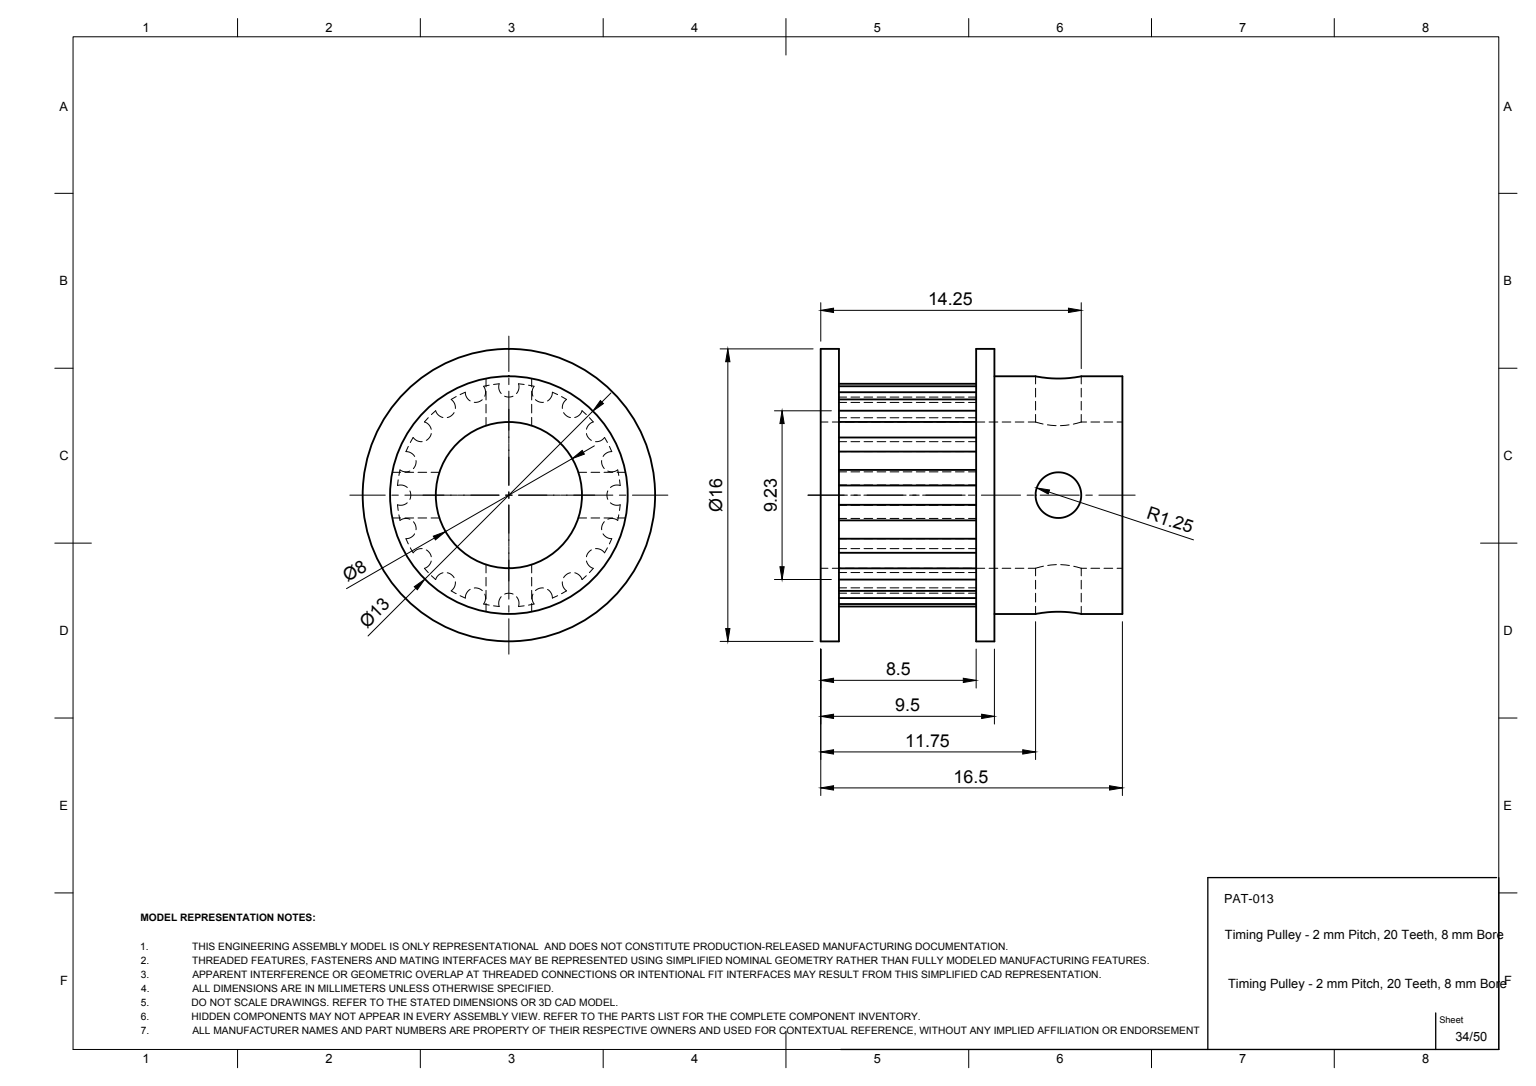
ISO-10303-21;
HEADER;
/* Generated by software containing ST-Developer
 * from STEP Tools, Inc. (www.steptools.com) 
 */

FILE_DESCRIPTION(
/* description */ ('Belt-driven linear axis on 2020 extrusion'),
/* implementation_level */ '2;1');

FILE_NAME(
/* name */ 'Timing Pulley - 2 mm Pitch, 20 Teeth, 8 mm Bore.step',
/* time_stamp */ '2026-10-28T03:26:09-07:00',
/* author */ (''),
/* organization */ (''),
/* preprocessor_version */ 'ST-DEVELOPER v20.2',
/* originating_system */ 'Autodesk Translation Framework v15.17.0.0',
/* authorisation */ '');

FILE_SCHEMA (('AUTOMOTIVE_DESIGN { 1 0 10303 214 3 1 1 }'));
ENDSEC;

DATA;
#10=MECHANICAL_DESIGN_GEOMETRIC_PRESENTATION_REPRESENTATION('',(#655),#20096);
#459=B_SPLINE_CURVE_WITH_KNOTS('',3,(#18624,#18625,#18626,#18627,#18628,
#18629,#18630,#18631,#18632,#18633),.UNSPECIFIED.,.F.,.F.,(4,2,2,2,4),(0.566550474129931,
0.613761886174531,0.66097329821913,0.708186965196186,0.755400632173242),
 .UNSPECIFIED.);
#460=B_SPLINE_CURVE_WITH_KNOTS('',3,(#18635,#18636,#18637,#18638,#18639,
#18640,#18641,#18642,#18643,#18644,#18645,#18646,#18647,#18648,#18649,#18650,
#18651,#18652),.UNSPECIFIED.,.F.,.F.,(4,2,2,2,2,2,2,2,4),(0.18885015804331,
0.23606157008791,0.283272982132509,0.330486649109565,0.377700316086621,
0.424913983063677,0.472127650040732,0.519339062085332,0.566550474129931),
 .UNSPECIFIED.);
#461=B_SPLINE_CURVE_WITH_KNOTS('',3,(#18653,#18654,#18655,#18656,#18657,
#18658,#18659,#18660,#18661,#18662),.UNSPECIFIED.,.F.,.F.,(4,2,2,2,4),(0.755400632173242,
0.802614299150298,0.849827966127353,0.897039378171953,0.944250790216552),
 .UNSPECIFIED.);
#462=B_SPLINE_CURVE_WITH_KNOTS('',3,(#18666,#18667,#18668,#18669,#18670,
#18671,#18672,#18673,#18674,#18675),.UNSPECIFIED.,.F.,.F.,(4,2,2,2,4),(0.189723673274825,
0.237146208024627,0.28456874277443,0.33200804466204,0.37944734654965),
 .UNSPECIFIED.);
#463=B_SPLINE_CURVE_WITH_KNOTS('',3,(#18677,#18678,#18679,#18680,#18681,
#18682,#18683,#18684,#18685,#18686),.UNSPECIFIED.,.F.,.F.,(4,2,2,2,4),(0.,
0.0474393018876097,0.0948786037752193,0.142301138525022,0.189723673274825),
 .UNSPECIFIED.);
#464=B_SPLINE_CURVE_WITH_KNOTS('',3,(#18688,#18689,#18690,#18691,#18692,
#18693,#18694,#18695,#18696,#18697),.UNSPECIFIED.,.F.,.F.,(4,2,2,2,4),(0.569171019824474,
0.616593554574277,0.66401608932408,0.711455391211689,0.758894693099299),
 .UNSPECIFIED.);
#465=B_SPLINE_CURVE_WITH_KNOTS('',3,(#18698,#18699,#18700,#18701,#18702,
#18703,#18704,#18705,#18706,#18707),.UNSPECIFIED.,.F.,.F.,(4,2,2,2,4),(0.37944734654965,
0.426886648437259,0.474325950324869,0.521748485074671,0.569171019824474),
 .UNSPECIFIED.);
#466=B_SPLINE_CURVE_WITH_KNOTS('',3,(#18711,#18712,#18713,#18714,#18715,
#18716,#18717,#18718,#18719,#18720,#18721,#18722,#18723,#18724,#18725,#18726,
#18727,#18728),.UNSPECIFIED.,.F.,.F.,(4,2,2,2,2,2,2,2,4),(0.,0.0474393018876097,
0.0948786037752194,0.142301138525022,0.189723673274825,0.237146208024628,
0.28456874277443,0.33200804466204,0.37944734654965),.UNSPECIFIED.);
#467=B_SPLINE_CURVE_WITH_KNOTS('',3,(#18729,#18730,#18731,#18732,#18733,
#18734,#18735,#18736,#18737,#18738,#18739,#18740,#18741,#18742,#18743,#18744,
#18745,#18746),.UNSPECIFIED.,.F.,.F.,(4,2,2,2,2,2,2,2,4),(0.37944734654965,
0.426886648437259,0.474325950324869,0.521748485074672,0.569171019824474,
0.616593554574277,0.66401608932408,0.711455391211689,0.758894693099299),
 .UNSPECIFIED.);
#468=B_SPLINE_CURVE_WITH_KNOTS('',3,(#18750,#18751,#18752,#18753,#18754,
#18755,#18756,#18757,#18758,#18759),.UNSPECIFIED.,.F.,.F.,(4,2,2,2,4),(0.566550474129931,
0.613761886174531,0.66097329821913,0.708186965196186,0.755400632173242),
 .UNSPECIFIED.);
#469=B_SPLINE_CURVE_WITH_KNOTS('',3,(#18761,#18762,#18763,#18764,#18765,
#18766,#18767,#18768,#18769,#18770,#18771,#18772,#18773,#18774,#18775,#18776,
#18777,#18778),.UNSPECIFIED.,.F.,.F.,(4,2,2,2,2,2,2,2,4),(0.188850158043311,
0.23606157008791,0.283272982132509,0.330486649109565,0.377700316086621,
0.424913983063677,0.472127650040733,0.519339062085332,0.566550474129931),
 .UNSPECIFIED.);
#470=B_SPLINE_CURVE_WITH_KNOTS('',3,(#18779,#18780,#18781,#18782,#18783,
#18784,#18785,#18786,#18787,#18788),.UNSPECIFIED.,.F.,.F.,(4,2,2,2,4),(0.755400632173242,
0.802614299150298,0.849827966127354,0.897039378171953,0.944250790216552),
 .UNSPECIFIED.);
#471=B_SPLINE_CURVE_WITH_KNOTS('',3,(#18798,#18799,#18800,#18801,#18802,
#18803,#18804,#18805,#18806,#18807,#18808,#18809,#18810,#18811,#18812,#18813,
#18814,#18815),.UNSPECIFIED.,.F.,.F.,(4,2,2,2,2,2,2,2,4),(0.18885015804331,
0.23606157008791,0.283272982132509,0.330486649109565,0.377700316086621,
0.424913983063677,0.472127650040732,0.519339062085332,0.566550474129931),
 .UNSPECIFIED.);
#472=B_SPLINE_CURVE_WITH_KNOTS('',3,(#18817,#18818,#18819,#18820,#18821,
#18822,#18823,#18824,#18825,#18826),.UNSPECIFIED.,.F.,.F.,(4,2,2,2,4),(0.566550474129931,
0.613761886174531,0.66097329821913,0.708186965196186,0.755400632173242),
 .UNSPECIFIED.);
#473=B_SPLINE_CURVE_WITH_KNOTS('',3,(#18827,#18828,#18829,#18830,#18831,
#18832,#18833,#18834,#18835,#18836),.UNSPECIFIED.,.F.,.F.,(4,2,2,2,4),(0.755400632173242,
0.802614299150298,0.849827966127353,0.897039378171953,0.944250790216552),
 .UNSPECIFIED.);
#474=B_SPLINE_CURVE_WITH_KNOTS('',3,(#18839,#18840,#18841,#18842,#18843,
#18844,#18845,#18846,#18847,#18848,#18849,#18850,#18851,#18852,#18853,#18854,
#18855,#18856),.UNSPECIFIED.,.F.,.F.,(4,2,2,2,2,2,2,2,4),(0.188850158043311,
0.23606157008791,0.283272982132509,0.330486649109565,0.377700316086621,
0.424913983063677,0.472127650040733,0.519339062085332,0.566550474129932),
 .UNSPECIFIED.);
#475=B_SPLINE_CURVE_WITH_KNOTS('',3,(#18858,#18859,#18860,#18861,#18862,
#18863,#18864,#18865,#18866,#18867),.UNSPECIFIED.,.F.,.F.,(4,2,2,2,4),(0.566550474129932,
0.613761886174531,0.66097329821913,0.708186965196186,0.755400632173242),
 .UNSPECIFIED.);
#476=B_SPLINE_CURVE_WITH_KNOTS('',3,(#18868,#18869,#18870,#18871,#18872,
#18873,#18874,#18875,#18876,#18877),.UNSPECIFIED.,.F.,.F.,(4,2,2,2,4),(0.755400632173242,
0.802614299150298,0.849827966127354,0.897039378171953,0.944250790216552),
 .UNSPECIFIED.);
#477=B_SPLINE_CURVE_WITH_KNOTS('',3,(#18882,#18883,#18884,#18885,#18886,
#18887,#18888,#18889,#18890,#18891,#18892,#18893,#18894,#18895,#18896,#18897,
#18898,#18899),.UNSPECIFIED.,.F.,.F.,(4,2,2,2,2,2,2,2,4),(0.,0.0474393018876097,
0.0948786037752193,0.142301138525022,0.189723673274825,0.237146208024627,
0.28456874277443,0.33200804466204,0.37944734654965),.UNSPECIFIED.);
#478=B_SPLINE_CURVE_WITH_KNOTS('',3,(#18900,#18901,#18902,#18903,#18904,
#18905,#18906,#18907,#18908,#18909,#18910,#18911,#18912,#18913,#18914,#18915,
#18916,#18917),.UNSPECIFIED.,.F.,.F.,(4,2,2,2,2,2,2,2,4),(0.37944734654965,
0.426886648437259,0.474325950324869,0.521748485074672,0.569171019824474,
0.616593554574277,0.66401608932408,0.711455391211689,0.758894693099299),
 .UNSPECIFIED.);
#479=B_SPLINE_CURVE_WITH_KNOTS('',3,(#18921,#18922,#18923,#18924,#18925,
#18926,#18927,#18928,#18929,#18930,#18931,#18932,#18933,#18934,#18935,#18936,
#18937,#18938),.UNSPECIFIED.,.F.,.F.,(4,2,2,2,2,2,2,2,4),(0.,0.0474393018876097,
0.0948786037752194,0.142301138525022,0.189723673274825,0.237146208024627,
0.28456874277443,0.33200804466204,0.37944734654965),.UNSPECIFIED.);
#480=B_SPLINE_CURVE_WITH_KNOTS('',3,(#18939,#18940,#18941,#18942,#18943,
#18944,#18945,#18946,#18947,#18948,#18949,#18950,#18951,#18952,#18953,#18954,
#18955,#18956),.UNSPECIFIED.,.F.,.F.,(4,2,2,2,2,2,2,2,4),(0.37944734654965,
0.426886648437259,0.474325950324869,0.521748485074672,0.569171019824474,
0.616593554574277,0.66401608932408,0.711455391211689,0.758894693099299),
 .UNSPECIFIED.);
#553=SHAPE_REPRESENTATION_RELATIONSHIP('SRR','None',#20352,#599);
#599=ADVANCED_BREP_SHAPE_REPRESENTATION('',(#710),#20083);
#655=STYLED_ITEM('',(#20664),#710);
#710=MANIFOLD_SOLID_BREP('Body1',#10969);
#851=FACE_BOUND('',#2438,.T.);
#852=FACE_BOUND('',#2439,.T.);
#853=FACE_BOUND('',#2440,.T.);
#854=FACE_BOUND('',#2444,.T.);
#855=FACE_BOUND('',#2445,.T.);
#856=FACE_BOUND('',#2446,.T.);
#857=FACE_BOUND('',#2448,.T.);
#858=FACE_BOUND('',#2450,.T.);
#859=FACE_BOUND('',#2453,.T.);
#860=FACE_BOUND('',#2455,.T.);
#861=FACE_BOUND('',#2458,.T.);
#1144=PLANE('',#12331);
#1145=PLANE('',#12332);
#1146=PLANE('',#12376);
#1147=PLANE('',#12377);
#1148=PLANE('',#12421);
#1680=FACE_OUTER_BOUND('',#2435,.T.);
#1681=FACE_OUTER_BOUND('',#2436,.T.);
#1682=FACE_OUTER_BOUND('',#2437,.T.);
#1683=FACE_OUTER_BOUND('',#2441,.T.);
#1684=FACE_OUTER_BOUND('',#2442,.T.);
#1685=FACE_OUTER_BOUND('',#2443,.T.);
#1686=FACE_OUTER_BOUND('',#2447,.T.);
#1687=FACE_OUTER_BOUND('',#2449,.T.);
#1688=FACE_OUTER_BOUND('',#2451,.T.);
#1689=FACE_OUTER_BOUND('',#2452,.T.);
#1690=FACE_OUTER_BOUND('',#2454,.T.);
#1691=FACE_OUTER_BOUND('',#2456,.T.);
#1692=FACE_OUTER_BOUND('',#2457,.T.);
#1693=FACE_OUTER_BOUND('',#2459,.T.);
#1694=FACE_OUTER_BOUND('',#2460,.T.);
#1695=FACE_OUTER_BOUND('',#2461,.T.);
#1696=FACE_OUTER_BOUND('',#2462,.T.);
#1697=FACE_OUTER_BOUND('',#2463,.T.);
#1698=FACE_OUTER_BOUND('',#2464,.T.);
#1699=FACE_OUTER_BOUND('',#2465,.T.);
#1700=FACE_OUTER_BOUND('',#2466,.T.);
#1701=FACE_OUTER_BOUND('',#2467,.T.);
#1702=FACE_OUTER_BOUND('',#2468,.T.);
#1703=FACE_OUTER_BOUND('',#2469,.T.);
#1704=FACE_OUTER_BOUND('',#2470,.T.);
#1705=FACE_OUTER_BOUND('',#2471,.T.);
#1706=FACE_OUTER_BOUND('',#2472,.T.);
#1707=FACE_OUTER_BOUND('',#2473,.T.);
#1708=FACE_OUTER_BOUND('',#2474,.T.);
#1709=FACE_OUTER_BOUND('',#2475,.T.);
#1710=FACE_OUTER_BOUND('',#2476,.T.);
#1711=FACE_OUTER_BOUND('',#2477,.T.);
#1712=FACE_OUTER_BOUND('',#2478,.T.);
#1713=FACE_OUTER_BOUND('',#2479,.T.);
#1714=FACE_OUTER_BOUND('',#2480,.T.);
#1715=FACE_OUTER_BOUND('',#2481,.T.);
#1716=FACE_OUTER_BOUND('',#2482,.T.);
#1717=FACE_OUTER_BOUND('',#2483,.T.);
#1718=FACE_OUTER_BOUND('',#2484,.T.);
#1719=FACE_OUTER_BOUND('',#2485,.T.);
#1720=FACE_OUTER_BOUND('',#2486,.T.);
#1721=FACE_OUTER_BOUND('',#2487,.T.);
#1722=FACE_OUTER_BOUND('',#2488,.T.);
#1723=FACE_OUTER_BOUND('',#2489,.T.);
#1724=FACE_OUTER_BOUND('',#2490,.T.);
#1725=FACE_OUTER_BOUND('',#2491,.T.);
#1726=FACE_OUTER_BOUND('',#2492,.T.);
#1727=FACE_OUTER_BOUND('',#2493,.T.);
#1728=FACE_OUTER_BOUND('',#2494,.T.);
#1729=FACE_OUTER_BOUND('',#2495,.T.);
#1730=FACE_OUTER_BOUND('',#2496,.T.);
#1731=FACE_OUTER_BOUND('',#2497,.T.);
#1732=FACE_OUTER_BOUND('',#2498,.T.);
#2435=EDGE_LOOP('',(#9133,#9134,#9135,#9136,#9137,#9138,#9139,#9140,#9141));
#2436=EDGE_LOOP('',(#9142,#9143,#9144,#9145,#9146,#9147,#9148));
#2437=EDGE_LOOP('',(#9149,#9150,#9151,#9152,#9153,#9154,#9155,#9156,#9157));
#2438=EDGE_LOOP('',(#9158,#9159,#9160));
#2439=EDGE_LOOP('',(#9161,#9162,#9163));
#2440=EDGE_LOOP('',(#9164,#9165,#9166));
#2441=EDGE_LOOP('',(#9167,#9168,#9169,#9170,#9171,#9172,#9173));
#2442=EDGE_LOOP('',(#9174,#9175,#9176,#9177,#9178,#9179,#9180));
#2443=EDGE_LOOP('',(#9181,#9182,#9183,#9184,#9185,#9186,#9187,#9188,#9189,
#9190));
#2444=EDGE_LOOP('',(#9191,#9192));
#2445=EDGE_LOOP('',(#9193,#9194));
#2446=EDGE_LOOP('',(#9195,#9196));
#2447=EDGE_LOOP('',(#9197));
#2448=EDGE_LOOP('',(#9198));
#2449=EDGE_LOOP('',(#9199));
#2450=EDGE_LOOP('',(#9200,#9201,#9202,#9203,#9204,#9205,#9206,#9207,#9208,
#9209,#9210,#9211,#9212,#9213,#9214,#9215,#9216,#9217,#9218,#9219,#9220,
#9221,#9222,#9223,#9224,#9225,#9226,#9227,#9228,#9229,#9230,#9231,#9232,
#9233,#9234,#9235,#9236,#9237,#9238,#9239));
#2451=EDGE_LOOP('',(#9240,#9241,#9242,#9243));
#2452=EDGE_LOOP('',(#9244));
#2453=EDGE_LOOP('',(#9245));
#2454=EDGE_LOOP('',(#9246));
#2455=EDGE_LOOP('',(#9247,#9248,#9249,#9250,#9251,#9252,#9253,#9254,#9255,
#9256,#9257,#9258,#9259,#9260,#9261,#9262,#9263,#9264,#9265,#9266,#9267,
#9268,#9269,#9270,#9271,#9272,#9273,#9274,#9275,#9276,#9277,#9278,#9279,
#9280,#9281,#9282,#9283,#9284,#9285,#9286));
#2456=EDGE_LOOP('',(#9287,#9288,#9289,#9290));
#2457=EDGE_LOOP('',(#9291));
#2458=EDGE_LOOP('',(#9292));
#2459=EDGE_LOOP('',(#9293,#9294,#9295,#9296));
#2460=EDGE_LOOP('',(#9297,#9298,#9299,#9300));
#2461=EDGE_LOOP('',(#9301,#9302,#9303,#9304));
#2462=EDGE_LOOP('',(#9305,#9306,#9307,#9308));
#2463=EDGE_LOOP('',(#9309,#9310,#9311,#9312));
#2464=EDGE_LOOP('',(#9313,#9314,#9315,#9316));
#2465=EDGE_LOOP('',(#9317,#9318,#9319,#9320));
#2466=EDGE_LOOP('',(#9321,#9322,#9323,#9324));
#2467=EDGE_LOOP('',(#9325,#9326,#9327,#9328));
#2468=EDGE_LOOP('',(#9329,#9330,#9331,#9332));
#2469=EDGE_LOOP('',(#9333,#9334,#9335,#9336));
#2470=EDGE_LOOP('',(#9337,#9338,#9339,#9340));
#2471=EDGE_LOOP('',(#9341,#9342,#9343,#9344));
#2472=EDGE_LOOP('',(#9345,#9346,#9347,#9348));
#2473=EDGE_LOOP('',(#9349,#9350,#9351,#9352));
#2474=EDGE_LOOP('',(#9353,#9354,#9355,#9356));
#2475=EDGE_LOOP('',(#9357,#9358,#9359,#9360));
#2476=EDGE_LOOP('',(#9361,#9362,#9363,#9364));
#2477=EDGE_LOOP('',(#9365,#9366,#9367,#9368));
#2478=EDGE_LOOP('',(#9369,#9370,#9371,#9372));
#2479=EDGE_LOOP('',(#9373,#9374,#9375,#9376));
#2480=EDGE_LOOP('',(#9377,#9378,#9379,#9380));
#2481=EDGE_LOOP('',(#9381,#9382,#9383,#9384));
#2482=EDGE_LOOP('',(#9385,#9386,#9387,#9388));
#2483=EDGE_LOOP('',(#9389,#9390,#9391,#9392));
#2484=EDGE_LOOP('',(#9393,#9394,#9395,#9396));
#2485=EDGE_LOOP('',(#9397,#9398,#9399,#9400));
#2486=EDGE_LOOP('',(#9401,#9402,#9403,#9404));
#2487=EDGE_LOOP('',(#9405,#9406,#9407,#9408));
#2488=EDGE_LOOP('',(#9409,#9410,#9411,#9412));
#2489=EDGE_LOOP('',(#9413,#9414,#9415,#9416));
#2490=EDGE_LOOP('',(#9417,#9418,#9419,#9420));
#2491=EDGE_LOOP('',(#9421,#9422,#9423,#9424));
#2492=EDGE_LOOP('',(#9425,#9426,#9427,#9428));
#2493=EDGE_LOOP('',(#9429,#9430,#9431,#9432));
#2494=EDGE_LOOP('',(#9433,#9434,#9435,#9436));
#2495=EDGE_LOOP('',(#9437,#9438,#9439,#9440));
#2496=EDGE_LOOP('',(#9441,#9442,#9443,#9444));
#2497=EDGE_LOOP('',(#9445,#9446,#9447,#9448));
#2498=EDGE_LOOP('',(#9449,#9450,#9451,#9452));
#3232=LINE('',#18664,#4089);
#3233=LINE('',#18748,#4090);
#3234=LINE('',#18792,#4091);
#3235=LINE('',#18794,#4092);
#3236=LINE('',#18880,#4093);
#3237=LINE('',#18957,#4094);
#3238=LINE('',#18961,#4095);
#3239=LINE('',#18963,#4096);
#3240=LINE('',#19052,#4097);
#3241=LINE('',#19140,#4098);
#3242=LINE('',#19143,#4099);
#3243=LINE('',#19144,#4100);
#3244=LINE('',#19146,#4101);
#3245=LINE('',#19148,#4102);
#3246=LINE('',#19150,#4103);
#3247=LINE('',#19152,#4104);
#3248=LINE('',#19154,#4105);
#3249=LINE('',#19156,#4106);
#3250=LINE('',#19158,#4107);
#3251=LINE('',#19160,#4108);
#3252=LINE('',#19162,#4109);
#3253=LINE('',#19164,#4110);
#3254=LINE('',#19166,#4111);
#3255=LINE('',#19168,#4112);
#3256=LINE('',#19170,#4113);
#3257=LINE('',#19172,#4114);
#3258=LINE('',#19174,#4115);
#3259=LINE('',#19176,#4116);
#3260=LINE('',#19178,#4117);
#3261=LINE('',#19180,#4118);
#3262=LINE('',#19182,#4119);
#3263=LINE('',#19184,#4120);
#3264=LINE('',#19186,#4121);
#3265=LINE('',#19188,#4122);
#3266=LINE('',#19190,#4123);
#3267=LINE('',#19192,#4124);
#3268=LINE('',#19194,#4125);
#3269=LINE('',#19196,#4126);
#3270=LINE('',#19198,#4127);
#3271=LINE('',#19200,#4128);
#3272=LINE('',#19202,#4129);
#3273=LINE('',#19204,#4130);
#3274=LINE('',#19206,#4131);
#3275=LINE('',#19208,#4132);
#3276=LINE('',#19210,#4133);
#3277=LINE('',#19212,#4134);
#3278=LINE('',#19214,#4135);
#3279=LINE('',#19216,#4136);
#3280=LINE('',#19218,#4137);
#3281=LINE('',#19220,#4138);
#4089=VECTOR('',#15016,0.125);
#4090=VECTOR('',#15019,0.125);
#4091=VECTOR('',#15024,0.65);
#4092=VECTOR('',#15025,0.65);
#4093=VECTOR('',#15030,0.125);
#4094=VECTOR('',#15033,0.125);
#4095=VECTOR('',#15038,0.4);
#4096=VECTOR('',#15039,0.4);
#4097=VECTOR('',#15132,0.8);
#4098=VECTOR('',#15223,0.8);
#4099=VECTOR('',#15228,1.);
#4100=VECTOR('',#15229,1.);
#4101=VECTOR('',#15232,1.);
#4102=VECTOR('',#15235,1.);
#4103=VECTOR('',#15238,1.);
#4104=VECTOR('',#15241,1.);
#4105=VECTOR('',#15244,1.);
#4106=VECTOR('',#15247,1.);
#4107=VECTOR('',#15250,1.);
#4108=VECTOR('',#15253,1.);
#4109=VECTOR('',#15256,1.);
#4110=VECTOR('',#15259,1.);
#4111=VECTOR('',#15262,1.);
#4112=VECTOR('',#15265,1.);
#4113=VECTOR('',#15268,1.);
#4114=VECTOR('',#15271,1.);
#4115=VECTOR('',#15274,1.);
#4116=VECTOR('',#15277,1.);
#4117=VECTOR('',#15280,1.);
#4118=VECTOR('',#15283,1.);
#4119=VECTOR('',#15286,1.);
#4120=VECTOR('',#15289,1.);
#4121=VECTOR('',#15292,1.);
#4122=VECTOR('',#15295,1.);
#4123=VECTOR('',#15298,1.);
#4124=VECTOR('',#15301,1.);
#4125=VECTOR('',#15304,1.);
#4126=VECTOR('',#15307,1.);
#4127=VECTOR('',#15310,1.);
#4128=VECTOR('',#15313,1.);
#4129=VECTOR('',#15316,1.);
#4130=VECTOR('',#15319,1.);
#4131=VECTOR('',#15322,1.);
#4132=VECTOR('',#15325,1.);
#4133=VECTOR('',#15328,1.);
#4134=VECTOR('',#15331,1.);
#4135=VECTOR('',#15334,1.);
#4136=VECTOR('',#15337,1.);
#4137=VECTOR('',#15340,1.);
#4138=VECTOR('',#15343,1.);
#4732=CIRCLE('',#12324,0.65);
#4733=CIRCLE('',#12325,0.65);
#4734=CIRCLE('',#12329,0.4);
#4735=CIRCLE('',#12330,0.4);
#4736=CIRCLE('',#12333,0.8);
#4737=CIRCLE('',#12334,0.0555);
#4738=CIRCLE('',#12335,0.611219772367581);
#4739=CIRCLE('',#12336,0.0555);
#4740=CIRCLE('',#12337,0.611219772367581);
#4741=CIRCLE('',#12338,0.0555);
#4742=CIRCLE('',#12339,0.611219772367581);
#4743=CIRCLE('',#12340,0.0555);
#4744=CIRCLE('',#12341,0.611219772367581);
#4745=CIRCLE('',#12342,0.0555);
#4746=CIRCLE('',#12343,0.611219772367581);
#4747=CIRCLE('',#12344,0.0555);
#4748=CIRCLE('',#12345,0.611219772367581);
#4749=CIRCLE('',#12346,0.0555);
#4750=CIRCLE('',#12347,0.611219772367581);
#4751=CIRCLE('',#12348,0.0555);
#4752=CIRCLE('',#12349,0.611219772367581);
#4753=CIRCLE('',#12350,0.0555);
#4754=CIRCLE('',#12351,0.611219772367581);
#4755=CIRCLE('',#12352,0.0555);
#4756=CIRCLE('',#12353,0.611219772367581);
#4757=CIRCLE('',#12354,0.0555);
#4758=CIRCLE('',#12355,0.611219772367581);
#4759=CIRCLE('',#12356,0.0555);
#4760=CIRCLE('',#12357,0.611219772367581);
#4761=CIRCLE('',#12358,0.0555);
#4762=CIRCLE('',#12359,0.611219772367581);
#4763=CIRCLE('',#12360,0.0555);
#4764=CIRCLE('',#12361,0.611219772367581);
#4765=CIRCLE('',#12362,0.0555);
#4766=CIRCLE('',#12363,0.611219772367581);
#4767=CIRCLE('',#12364,0.0555);
#4768=CIRCLE('',#12365,0.611219772367581);
#4769=CIRCLE('',#12366,0.0555);
#4770=CIRCLE('',#12367,0.611219772367581);
#4771=CIRCLE('',#12368,0.0555);
#4772=CIRCLE('',#12369,0.611219772367581);
#4773=CIRCLE('',#12370,0.0555);
#4774=CIRCLE('',#12371,0.611219772367581);
#4775=CIRCLE('',#12372,0.0555);
#4776=CIRCLE('',#12373,0.611219772367581);
#4777=CIRCLE('',#12375,0.8);
#4778=CIRCLE('',#12378,0.8);
#4779=CIRCLE('',#12379,0.0555);
#4780=CIRCLE('',#12380,0.611219772367581);
#4781=CIRCLE('',#12381,0.0555);
#4782=CIRCLE('',#12382,0.611219772367581);
#4783=CIRCLE('',#12383,0.0555);
#4784=CIRCLE('',#12384,0.611219772367581);
#4785=CIRCLE('',#12385,0.0555);
#4786=CIRCLE('',#12386,0.611219772367581);
#4787=CIRCLE('',#12387,0.0555);
#4788=CIRCLE('',#12388,0.611219772367581);
#4789=CIRCLE('',#12389,0.0555);
#4790=CIRCLE('',#12390,0.611219772367581);
#4791=CIRCLE('',#12391,0.0555);
#4792=CIRCLE('',#12392,0.611219772367581);
#4793=CIRCLE('',#12393,0.0555);
#4794=CIRCLE('',#12394,0.611219772367581);
#4795=CIRCLE('',#12395,0.0555);
#4796=CIRCLE('',#12396,0.611219772367581);
#4797=CIRCLE('',#12397,0.0555);
#4798=CIRCLE('',#12398,0.611219772367581);
#4799=CIRCLE('',#12399,0.0555);
#4800=CIRCLE('',#12400,0.611219772367581);
#4801=CIRCLE('',#12401,0.0555);
#4802=CIRCLE('',#12402,0.611219772367581);
#4803=CIRCLE('',#12403,0.0555);
#4804=CIRCLE('',#12404,0.611219772367581);
#4805=CIRCLE('',#12405,0.0555);
#4806=CIRCLE('',#12406,0.611219772367581);
#4807=CIRCLE('',#12407,0.0555);
#4808=CIRCLE('',#12408,0.611219772367581);
#4809=CIRCLE('',#12409,0.0555);
#4810=CIRCLE('',#12410,0.611219772367581);
#4811=CIRCLE('',#12411,0.0555);
#4812=CIRCLE('',#12412,0.611219772367581);
#4813=CIRCLE('',#12413,0.0555);
#4814=CIRCLE('',#12414,0.611219772367581);
#4815=CIRCLE('',#12415,0.0555);
#4816=CIRCLE('',#12416,0.611219772367581);
#4817=CIRCLE('',#12417,0.0555);
#4818=CIRCLE('',#12418,0.611219772367581);
#4819=CIRCLE('',#12420,0.8);
#5527=VERTEX_POINT('',#18622);
#5528=VERTEX_POINT('',#18623);
#5529=VERTEX_POINT('',#18634);
#5530=VERTEX_POINT('',#18663);
#5531=VERTEX_POINT('',#18665);
#5532=VERTEX_POINT('',#18676);
#5533=VERTEX_POINT('',#18687);
#5534=VERTEX_POINT('',#18709);
#5535=VERTEX_POINT('',#18710);
#5536=VERTEX_POINT('',#18747);
#5537=VERTEX_POINT('',#18749);
#5538=VERTEX_POINT('',#18760);
#5539=VERTEX_POINT('',#18790);
#5540=VERTEX_POINT('',#18793);
#5541=VERTEX_POINT('',#18796);
#5542=VERTEX_POINT('',#18797);
#5543=VERTEX_POINT('',#18816);
#5544=VERTEX_POINT('',#18837);
#5545=VERTEX_POINT('',#18838);
#5546=VERTEX_POINT('',#18857);
#5547=VERTEX_POINT('',#18879);
#5548=VERTEX_POINT('',#18881);
#5549=VERTEX_POINT('',#18919);
#5550=VERTEX_POINT('',#18920);
#5551=VERTEX_POINT('',#18959);
#5552=VERTEX_POINT('',#18962);
#5553=VERTEX_POINT('',#18967);
#5554=VERTEX_POINT('',#18969);
#5555=VERTEX_POINT('',#18970);
#5556=VERTEX_POINT('',#18972);
#5557=VERTEX_POINT('',#18974);
#5558=VERTEX_POINT('',#18976);
#5559=VERTEX_POINT('',#18978);
#5560=VERTEX_POINT('',#18980);
#5561=VERTEX_POINT('',#18982);
#5562=VERTEX_POINT('',#18984);
#5563=VERTEX_POINT('',#18986);
#5564=VERTEX_POINT('',#18988);
#5565=VERTEX_POINT('',#18990);
#5566=VERTEX_POINT('',#18992);
#5567=VERTEX_POINT('',#18994);
#5568=VERTEX_POINT('',#18996);
#5569=VERTEX_POINT('',#18998);
#5570=VERTEX_POINT('',#19000);
#5571=VERTEX_POINT('',#19002);
#5572=VERTEX_POINT('',#19004);
#5573=VERTEX_POINT('',#19006);
#5574=VERTEX_POINT('',#19008);
#5575=VERTEX_POINT('',#19010);
#5576=VERTEX_POINT('',#19012);
#5577=VERTEX_POINT('',#19014);
#5578=VERTEX_POINT('',#19016);
#5579=VERTEX_POINT('',#19018);
#5580=VERTEX_POINT('',#19020);
#5581=VERTEX_POINT('',#19022);
#5582=VERTEX_POINT('',#19024);
#5583=VERTEX_POINT('',#19026);
#5584=VERTEX_POINT('',#19028);
#5585=VERTEX_POINT('',#19030);
#5586=VERTEX_POINT('',#19032);
#5587=VERTEX_POINT('',#19034);
#5588=VERTEX_POINT('',#19036);
#5589=VERTEX_POINT('',#19038);
#5590=VERTEX_POINT('',#19040);
#5591=VERTEX_POINT('',#19042);
#5592=VERTEX_POINT('',#19044);
#5593=VERTEX_POINT('',#19046);
#5594=VERTEX_POINT('',#19050);
#5595=VERTEX_POINT('',#19055);
#5596=VERTEX_POINT('',#19057);
#5597=VERTEX_POINT('',#19058);
#5598=VERTEX_POINT('',#19060);
#5599=VERTEX_POINT('',#19062);
#5600=VERTEX_POINT('',#19064);
#5601=VERTEX_POINT('',#19066);
#5602=VERTEX_POINT('',#19068);
#5603=VERTEX_POINT('',#19070);
#5604=VERTEX_POINT('',#19072);
#5605=VERTEX_POINT('',#19074);
#5606=VERTEX_POINT('',#19076);
#5607=VERTEX_POINT('',#19078);
#5608=VERTEX_POINT('',#19080);
#5609=VERTEX_POINT('',#19082);
#5610=VERTEX_POINT('',#19084);
#5611=VERTEX_POINT('',#19086);
#5612=VERTEX_POINT('',#19088);
#5613=VERTEX_POINT('',#19090);
#5614=VERTEX_POINT('',#19092);
#5615=VERTEX_POINT('',#19094);
#5616=VERTEX_POINT('',#19096);
#5617=VERTEX_POINT('',#19098);
#5618=VERTEX_POINT('',#19100);
#5619=VERTEX_POINT('',#19102);
#5620=VERTEX_POINT('',#19104);
#5621=VERTEX_POINT('',#19106);
#5622=VERTEX_POINT('',#19108);
#5623=VERTEX_POINT('',#19110);
#5624=VERTEX_POINT('',#19112);
#5625=VERTEX_POINT('',#19114);
#5626=VERTEX_POINT('',#19116);
#5627=VERTEX_POINT('',#19118);
#5628=VERTEX_POINT('',#19120);
#5629=VERTEX_POINT('',#19122);
#5630=VERTEX_POINT('',#19124);
#5631=VERTEX_POINT('',#19126);
#5632=VERTEX_POINT('',#19128);
#5633=VERTEX_POINT('',#19130);
#5634=VERTEX_POINT('',#19132);
#5635=VERTEX_POINT('',#19134);
#5636=VERTEX_POINT('',#19138);
#6781=EDGE_CURVE('',#5527,#5528,#459,.T.);
#6782=EDGE_CURVE('',#5529,#5527,#460,.T.);
#6783=EDGE_CURVE('',#5528,#5529,#461,.T.);
#6784=EDGE_CURVE('',#5528,#5530,#3232,.T.);
#6785=EDGE_CURVE('',#5531,#5530,#462,.T.);
#6786=EDGE_CURVE('',#5532,#5531,#463,.T.);
#6787=EDGE_CURVE('',#5533,#5532,#464,.T.);
#6788=EDGE_CURVE('',#5530,#5533,#465,.T.);
#6789=EDGE_CURVE('',#5534,#5535,#466,.T.);
#6790=EDGE_CURVE('',#5535,#5534,#467,.T.);
#6791=EDGE_CURVE('',#5535,#5536,#3233,.T.);
#6792=EDGE_CURVE('',#5537,#5536,#468,.T.);
#6793=EDGE_CURVE('',#5538,#5537,#469,.T.);
#6794=EDGE_CURVE('',#5536,#5538,#470,.T.);
#6795=EDGE_CURVE('',#5539,#5539,#4732,.T.);
#6796=EDGE_CURVE('',#5539,#5529,#3234,.T.);
#6797=EDGE_CURVE('',#5527,#5540,#3235,.T.);
#6798=EDGE_CURVE('',#5540,#5540,#4733,.T.);
#6799=EDGE_CURVE('',#5541,#5542,#471,.T.);
#6800=EDGE_CURVE('',#5542,#5543,#472,.T.);
#6801=EDGE_CURVE('',#5543,#5541,#473,.T.);
#6802=EDGE_CURVE('',#5544,#5545,#474,.T.);
#6803=EDGE_CURVE('',#5545,#5546,#475,.T.);
#6804=EDGE_CURVE('',#5546,#5544,#476,.T.);
#6805=EDGE_CURVE('',#5543,#5547,#3236,.T.);
#6806=EDGE_CURVE('',#5548,#5547,#477,.T.);
#6807=EDGE_CURVE('',#5547,#5548,#478,.T.);
#6808=EDGE_CURVE('',#5549,#5550,#479,.T.);
#6809=EDGE_CURVE('',#5550,#5549,#480,.T.);
#6810=EDGE_CURVE('',#5550,#5546,#3237,.T.);
#6811=EDGE_CURVE('',#5551,#5551,#4734,.T.);
#6812=EDGE_CURVE('',#5551,#5531,#3238,.T.);
#6813=EDGE_CURVE('',#5533,#5552,#3239,.T.);
#6814=EDGE_CURVE('',#5552,#5552,#4735,.T.);
#6815=EDGE_CURVE('',#5553,#5553,#4736,.T.);
#6816=EDGE_CURVE('',#5554,#5555,#4737,.T.);
#6817=EDGE_CURVE('',#5556,#5555,#4738,.T.);
#6818=EDGE_CURVE('',#5556,#5557,#4739,.T.);
#6819=EDGE_CURVE('',#5558,#5557,#4740,.T.);
#6820=EDGE_CURVE('',#5558,#5559,#4741,.T.);
#6821=EDGE_CURVE('',#5560,#5559,#4742,.T.);
#6822=EDGE_CURVE('',#5560,#5561,#4743,.T.);
#6823=EDGE_CURVE('',#5562,#5561,#4744,.T.);
#6824=EDGE_CURVE('',#5562,#5563,#4745,.T.);
#6825=EDGE_CURVE('',#5564,#5563,#4746,.T.);
#6826=EDGE_CURVE('',#5564,#5565,#4747,.T.);
#6827=EDGE_CURVE('',#5566,#5565,#4748,.T.);
#6828=EDGE_CURVE('',#5566,#5567,#4749,.T.);
#6829=EDGE_CURVE('',#5568,#5567,#4750,.T.);
#6830=EDGE_CURVE('',#5568,#5569,#4751,.T.);
#6831=EDGE_CURVE('',#5570,#5569,#4752,.T.);
#6832=EDGE_CURVE('',#5570,#5571,#4753,.T.);
#6833=EDGE_CURVE('',#5572,#5571,#4754,.T.);
#6834=EDGE_CURVE('',#5572,#5573,#4755,.T.);
#6835=EDGE_CURVE('',#5574,#5573,#4756,.T.);
#6836=EDGE_CURVE('',#5574,#5575,#4757,.T.);
#6837=EDGE_CURVE('',#5576,#5575,#4758,.T.);
#6838=EDGE_CURVE('',#5576,#5577,#4759,.T.);
#6839=EDGE_CURVE('',#5578,#5577,#4760,.T.);
#6840=EDGE_CURVE('',#5578,#5579,#4761,.T.);
#6841=EDGE_CURVE('',#5580,#5579,#4762,.T.);
#6842=EDGE_CURVE('',#5580,#5581,#4763,.T.);
#6843=EDGE_CURVE('',#5582,#5581,#4764,.T.);
#6844=EDGE_CURVE('',#5582,#5583,#4765,.T.);
#6845=EDGE_CURVE('',#5584,#5583,#4766,.T.);
#6846=EDGE_CURVE('',#5584,#5585,#4767,.T.);
#6847=EDGE_CURVE('',#5586,#5585,#4768,.T.);
#6848=EDGE_CURVE('',#5586,#5587,#4769,.T.);
#6849=EDGE_CURVE('',#5588,#5587,#4770,.T.);
#6850=EDGE_CURVE('',#5588,#5589,#4771,.T.);
#6851=EDGE_CURVE('',#5590,#5589,#4772,.T.);
#6852=EDGE_CURVE('',#5590,#5591,#4773,.T.);
#6853=EDGE_CURVE('',#5592,#5591,#4774,.T.);
#6854=EDGE_CURVE('',#5592,#5593,#4775,.T.);
#6855=EDGE_CURVE('',#5554,#5593,#4776,.T.);
#6856=EDGE_CURVE('',#5594,#5594,#4777,.T.);
#6857=EDGE_CURVE('',#5594,#5553,#3240,.T.);
#6858=EDGE_CURVE('',#5595,#5595,#4778,.T.);
#6859=EDGE_CURVE('',#5596,#5597,#4779,.T.);
#6860=EDGE_CURVE('',#5597,#5598,#4780,.T.);
#6861=EDGE_CURVE('',#5598,#5599,#4781,.T.);
#6862=EDGE_CURVE('',#5599,#5600,#4782,.T.);
#6863=EDGE_CURVE('',#5600,#5601,#4783,.T.);
#6864=EDGE_CURVE('',#5601,#5602,#4784,.T.);
#6865=EDGE_CURVE('',#5602,#5603,#4785,.T.);
#6866=EDGE_CURVE('',#5603,#5604,#4786,.T.);
#6867=EDGE_CURVE('',#5604,#5605,#4787,.T.);
#6868=EDGE_CURVE('',#5605,#5606,#4788,.T.);
#6869=EDGE_CURVE('',#5606,#5607,#4789,.T.);
#6870=EDGE_CURVE('',#5607,#5608,#4790,.T.);
#6871=EDGE_CURVE('',#5608,#5609,#4791,.T.);
#6872=EDGE_CURVE('',#5609,#5610,#4792,.T.);
#6873=EDGE_CURVE('',#5610,#5611,#4793,.T.);
#6874=EDGE_CURVE('',#5611,#5612,#4794,.T.);
#6875=EDGE_CURVE('',#5612,#5613,#4795,.T.);
#6876=EDGE_CURVE('',#5613,#5614,#4796,.T.);
#6877=EDGE_CURVE('',#5614,#5615,#4797,.T.);
#6878=EDGE_CURVE('',#5615,#5616,#4798,.T.);
#6879=EDGE_CURVE('',#5616,#5617,#4799,.T.);
#6880=EDGE_CURVE('',#5617,#5618,#4800,.T.);
#6881=EDGE_CURVE('',#5618,#5619,#4801,.T.);
#6882=EDGE_CURVE('',#5619,#5620,#4802,.T.);
#6883=EDGE_CURVE('',#5620,#5621,#4803,.T.);
#6884=EDGE_CURVE('',#5621,#5622,#4804,.T.);
#6885=EDGE_CURVE('',#5622,#5623,#4805,.T.);
#6886=EDGE_CURVE('',#5623,#5624,#4806,.T.);
#6887=EDGE_CURVE('',#5624,#5625,#4807,.T.);
#6888=EDGE_CURVE('',#5625,#5626,#4808,.T.);
#6889=EDGE_CURVE('',#5626,#5627,#4809,.T.);
#6890=EDGE_CURVE('',#5627,#5628,#4810,.T.);
#6891=EDGE_CURVE('',#5628,#5629,#4811,.T.);
#6892=EDGE_CURVE('',#5629,#5630,#4812,.T.);
#6893=EDGE_CURVE('',#5630,#5631,#4813,.T.);
#6894=EDGE_CURVE('',#5631,#5632,#4814,.T.);
#6895=EDGE_CURVE('',#5632,#5633,#4815,.T.);
#6896=EDGE_CURVE('',#5633,#5634,#4816,.T.);
#6897=EDGE_CURVE('',#5634,#5635,#4817,.T.);
#6898=EDGE_CURVE('',#5635,#5596,#4818,.T.);
#6899=EDGE_CURVE('',#5636,#5636,#4819,.T.);
#6900=EDGE_CURVE('',#5636,#5595,#3241,.T.);
#6901=EDGE_CURVE('',#5597,#5554,#3242,.T.);
#6902=EDGE_CURVE('',#5555,#5596,#3243,.T.);
#6903=EDGE_CURVE('',#5635,#5556,#3244,.T.);
#6904=EDGE_CURVE('',#5557,#5634,#3245,.T.);
#6905=EDGE_CURVE('',#5633,#5558,#3246,.T.);
#6906=EDGE_CURVE('',#5559,#5632,#3247,.T.);
#6907=EDGE_CURVE('',#5631,#5560,#3248,.T.);
#6908=EDGE_CURVE('',#5561,#5630,#3249,.T.);
#6909=EDGE_CURVE('',#5629,#5562,#3250,.T.);
#6910=EDGE_CURVE('',#5563,#5628,#3251,.T.);
#6911=EDGE_CURVE('',#5627,#5564,#3252,.T.);
#6912=EDGE_CURVE('',#5565,#5626,#3253,.T.);
#6913=EDGE_CURVE('',#5625,#5566,#3254,.T.);
#6914=EDGE_CURVE('',#5567,#5624,#3255,.T.);
#6915=EDGE_CURVE('',#5623,#5568,#3256,.T.);
#6916=EDGE_CURVE('',#5569,#5622,#3257,.T.);
#6917=EDGE_CURVE('',#5621,#5570,#3258,.T.);
#6918=EDGE_CURVE('',#5571,#5620,#3259,.T.);
#6919=EDGE_CURVE('',#5619,#5572,#3260,.T.);
#6920=EDGE_CURVE('',#5573,#5618,#3261,.T.);
#6921=EDGE_CURVE('',#5617,#5574,#3262,.T.);
#6922=EDGE_CURVE('',#5575,#5616,#3263,.T.);
#6923=EDGE_CURVE('',#5615,#5576,#3264,.T.);
#6924=EDGE_CURVE('',#5577,#5614,#3265,.T.);
#6925=EDGE_CURVE('',#5613,#5578,#3266,.T.);
#6926=EDGE_CURVE('',#5579,#5612,#3267,.T.);
#6927=EDGE_CURVE('',#5611,#5580,#3268,.T.);
#6928=EDGE_CURVE('',#5581,#5610,#3269,.T.);
#6929=EDGE_CURVE('',#5609,#5582,#3270,.T.);
#6930=EDGE_CURVE('',#5583,#5608,#3271,.T.);
#6931=EDGE_CURVE('',#5607,#5584,#3272,.T.);
#6932=EDGE_CURVE('',#5585,#5606,#3273,.T.);
#6933=EDGE_CURVE('',#5605,#5586,#3274,.T.);
#6934=EDGE_CURVE('',#5587,#5604,#3275,.T.);
#6935=EDGE_CURVE('',#5603,#5588,#3276,.T.);
#6936=EDGE_CURVE('',#5589,#5602,#3277,.T.);
#6937=EDGE_CURVE('',#5601,#5590,#3278,.T.);
#6938=EDGE_CURVE('',#5591,#5600,#3279,.T.);
#6939=EDGE_CURVE('',#5593,#5598,#3280,.T.);
#6940=EDGE_CURVE('',#5599,#5592,#3281,.T.);
#9133=ORIENTED_EDGE('',*,*,#6781,.F.);
#9134=ORIENTED_EDGE('',*,*,#6782,.F.);
#9135=ORIENTED_EDGE('',*,*,#6783,.F.);
#9136=ORIENTED_EDGE('',*,*,#6784,.T.);
#9137=ORIENTED_EDGE('',*,*,#6785,.F.);
#9138=ORIENTED_EDGE('',*,*,#6786,.F.);
#9139=ORIENTED_EDGE('',*,*,#6787,.F.);
#9140=ORIENTED_EDGE('',*,*,#6788,.F.);
#9141=ORIENTED_EDGE('',*,*,#6784,.F.);
#9142=ORIENTED_EDGE('',*,*,#6789,.F.);
#9143=ORIENTED_EDGE('',*,*,#6790,.F.);
#9144=ORIENTED_EDGE('',*,*,#6791,.T.);
#9145=ORIENTED_EDGE('',*,*,#6792,.F.);
#9146=ORIENTED_EDGE('',*,*,#6793,.F.);
#9147=ORIENTED_EDGE('',*,*,#6794,.F.);
#9148=ORIENTED_EDGE('',*,*,#6791,.F.);
#9149=ORIENTED_EDGE('',*,*,#6795,.F.);
#9150=ORIENTED_EDGE('',*,*,#6796,.T.);
#9151=ORIENTED_EDGE('',*,*,#6782,.T.);
#9152=ORIENTED_EDGE('',*,*,#6797,.T.);
#9153=ORIENTED_EDGE('',*,*,#6798,.F.);
#9154=ORIENTED_EDGE('',*,*,#6797,.F.);
#9155=ORIENTED_EDGE('',*,*,#6781,.T.);
#9156=ORIENTED_EDGE('',*,*,#6783,.T.);
#9157=ORIENTED_EDGE('',*,*,#6796,.F.);
#9158=ORIENTED_EDGE('',*,*,#6793,.T.);
#9159=ORIENTED_EDGE('',*,*,#6792,.T.);
#9160=ORIENTED_EDGE('',*,*,#6794,.T.);
#9161=ORIENTED_EDGE('',*,*,#6799,.T.);
#9162=ORIENTED_EDGE('',*,*,#6800,.T.);
#9163=ORIENTED_EDGE('',*,*,#6801,.T.);
#9164=ORIENTED_EDGE('',*,*,#6802,.T.);
#9165=ORIENTED_EDGE('',*,*,#6803,.T.);
#9166=ORIENTED_EDGE('',*,*,#6804,.T.);
#9167=ORIENTED_EDGE('',*,*,#6800,.F.);
#9168=ORIENTED_EDGE('',*,*,#6799,.F.);
#9169=ORIENTED_EDGE('',*,*,#6801,.F.);
#9170=ORIENTED_EDGE('',*,*,#6805,.T.);
#9171=ORIENTED_EDGE('',*,*,#6806,.F.);
#9172=ORIENTED_EDGE('',*,*,#6807,.F.);
#9173=ORIENTED_EDGE('',*,*,#6805,.F.);
#9174=ORIENTED_EDGE('',*,*,#6808,.F.);
#9175=ORIENTED_EDGE('',*,*,#6809,.F.);
#9176=ORIENTED_EDGE('',*,*,#6810,.T.);
#9177=ORIENTED_EDGE('',*,*,#6803,.F.);
#9178=ORIENTED_EDGE('',*,*,#6802,.F.);
#9179=ORIENTED_EDGE('',*,*,#6804,.F.);
#9180=ORIENTED_EDGE('',*,*,#6810,.F.);
#9181=ORIENTED_EDGE('',*,*,#6811,.F.);
#9182=ORIENTED_EDGE('',*,*,#6812,.T.);
#9183=ORIENTED_EDGE('',*,*,#6785,.T.);
#9184=ORIENTED_EDGE('',*,*,#6788,.T.);
#9185=ORIENTED_EDGE('',*,*,#6813,.T.);
#9186=ORIENTED_EDGE('',*,*,#6814,.F.);
#9187=ORIENTED_EDGE('',*,*,#6813,.F.);
#9188=ORIENTED_EDGE('',*,*,#6787,.T.);
#9189=ORIENTED_EDGE('',*,*,#6786,.T.);
#9190=ORIENTED_EDGE('',*,*,#6812,.F.);
#9191=ORIENTED_EDGE('',*,*,#6789,.T.);
#9192=ORIENTED_EDGE('',*,*,#6790,.T.);
#9193=ORIENTED_EDGE('',*,*,#6808,.T.);
#9194=ORIENTED_EDGE('',*,*,#6809,.T.);
#9195=ORIENTED_EDGE('',*,*,#6806,.T.);
#9196=ORIENTED_EDGE('',*,*,#6807,.T.);
#9197=ORIENTED_EDGE('',*,*,#6795,.T.);
#9198=ORIENTED_EDGE('',*,*,#6811,.T.);
#9199=ORIENTED_EDGE('',*,*,#6815,.T.);
#9200=ORIENTED_EDGE('',*,*,#6816,.T.);
#9201=ORIENTED_EDGE('',*,*,#6817,.F.);
#9202=ORIENTED_EDGE('',*,*,#6818,.T.);
#9203=ORIENTED_EDGE('',*,*,#6819,.F.);
#9204=ORIENTED_EDGE('',*,*,#6820,.T.);
#9205=ORIENTED_EDGE('',*,*,#6821,.F.);
#9206=ORIENTED_EDGE('',*,*,#6822,.T.);
#9207=ORIENTED_EDGE('',*,*,#6823,.F.);
#9208=ORIENTED_EDGE('',*,*,#6824,.T.);
#9209=ORIENTED_EDGE('',*,*,#6825,.F.);
#9210=ORIENTED_EDGE('',*,*,#6826,.T.);
#9211=ORIENTED_EDGE('',*,*,#6827,.F.);
#9212=ORIENTED_EDGE('',*,*,#6828,.T.);
#9213=ORIENTED_EDGE('',*,*,#6829,.F.);
#9214=ORIENTED_EDGE('',*,*,#6830,.T.);
#9215=ORIENTED_EDGE('',*,*,#6831,.F.);
#9216=ORIENTED_EDGE('',*,*,#6832,.T.);
#9217=ORIENTED_EDGE('',*,*,#6833,.F.);
#9218=ORIENTED_EDGE('',*,*,#6834,.T.);
#9219=ORIENTED_EDGE('',*,*,#6835,.F.);
#9220=ORIENTED_EDGE('',*,*,#6836,.T.);
#9221=ORIENTED_EDGE('',*,*,#6837,.F.);
#9222=ORIENTED_EDGE('',*,*,#6838,.T.);
#9223=ORIENTED_EDGE('',*,*,#6839,.F.);
#9224=ORIENTED_EDGE('',*,*,#6840,.T.);
#9225=ORIENTED_EDGE('',*,*,#6841,.F.);
#9226=ORIENTED_EDGE('',*,*,#6842,.T.);
#9227=ORIENTED_EDGE('',*,*,#6843,.F.);
#9228=ORIENTED_EDGE('',*,*,#6844,.T.);
#9229=ORIENTED_EDGE('',*,*,#6845,.F.);
#9230=ORIENTED_EDGE('',*,*,#6846,.T.);
#9231=ORIENTED_EDGE('',*,*,#6847,.F.);
#9232=ORIENTED_EDGE('',*,*,#6848,.T.);
#9233=ORIENTED_EDGE('',*,*,#6849,.F.);
#9234=ORIENTED_EDGE('',*,*,#6850,.T.);
#9235=ORIENTED_EDGE('',*,*,#6851,.F.);
#9236=ORIENTED_EDGE('',*,*,#6852,.T.);
#9237=ORIENTED_EDGE('',*,*,#6853,.F.);
#9238=ORIENTED_EDGE('',*,*,#6854,.T.);
#9239=ORIENTED_EDGE('',*,*,#6855,.F.);
#9240=ORIENTED_EDGE('',*,*,#6856,.F.);
#9241=ORIENTED_EDGE('',*,*,#6857,.T.);
#9242=ORIENTED_EDGE('',*,*,#6815,.F.);
#9243=ORIENTED_EDGE('',*,*,#6857,.F.);
#9244=ORIENTED_EDGE('',*,*,#6856,.T.);
#9245=ORIENTED_EDGE('',*,*,#6798,.T.);
#9246=ORIENTED_EDGE('',*,*,#6858,.F.);
#9247=ORIENTED_EDGE('',*,*,#6859,.T.);
#9248=ORIENTED_EDGE('',*,*,#6860,.T.);
#9249=ORIENTED_EDGE('',*,*,#6861,.T.);
#9250=ORIENTED_EDGE('',*,*,#6862,.T.);
#9251=ORIENTED_EDGE('',*,*,#6863,.T.);
#9252=ORIENTED_EDGE('',*,*,#6864,.T.);
#9253=ORIENTED_EDGE('',*,*,#6865,.T.);
#9254=ORIENTED_EDGE('',*,*,#6866,.T.);
#9255=ORIENTED_EDGE('',*,*,#6867,.T.);
#9256=ORIENTED_EDGE('',*,*,#6868,.T.);
#9257=ORIENTED_EDGE('',*,*,#6869,.T.);
#9258=ORIENTED_EDGE('',*,*,#6870,.T.);
#9259=ORIENTED_EDGE('',*,*,#6871,.T.);
#9260=ORIENTED_EDGE('',*,*,#6872,.T.);
#9261=ORIENTED_EDGE('',*,*,#6873,.T.);
#9262=ORIENTED_EDGE('',*,*,#6874,.T.);
#9263=ORIENTED_EDGE('',*,*,#6875,.T.);
#9264=ORIENTED_EDGE('',*,*,#6876,.T.);
#9265=ORIENTED_EDGE('',*,*,#6877,.T.);
#9266=ORIENTED_EDGE('',*,*,#6878,.T.);
#9267=ORIENTED_EDGE('',*,*,#6879,.T.);
#9268=ORIENTED_EDGE('',*,*,#6880,.T.);
#9269=ORIENTED_EDGE('',*,*,#6881,.T.);
#9270=ORIENTED_EDGE('',*,*,#6882,.T.);
#9271=ORIENTED_EDGE('',*,*,#6883,.T.);
#9272=ORIENTED_EDGE('',*,*,#6884,.T.);
#9273=ORIENTED_EDGE('',*,*,#6885,.T.);
#9274=ORIENTED_EDGE('',*,*,#6886,.T.);
#9275=ORIENTED_EDGE('',*,*,#6887,.T.);
#9276=ORIENTED_EDGE('',*,*,#6888,.T.);
#9277=ORIENTED_EDGE('',*,*,#6889,.T.);
#9278=ORIENTED_EDGE('',*,*,#6890,.T.);
#9279=ORIENTED_EDGE('',*,*,#6891,.T.);
#9280=ORIENTED_EDGE('',*,*,#6892,.T.);
#9281=ORIENTED_EDGE('',*,*,#6893,.T.);
#9282=ORIENTED_EDGE('',*,*,#6894,.T.);
#9283=ORIENTED_EDGE('',*,*,#6895,.T.);
#9284=ORIENTED_EDGE('',*,*,#6896,.T.);
#9285=ORIENTED_EDGE('',*,*,#6897,.T.);
#9286=ORIENTED_EDGE('',*,*,#6898,.T.);
#9287=ORIENTED_EDGE('',*,*,#6899,.F.);
#9288=ORIENTED_EDGE('',*,*,#6900,.T.);
#9289=ORIENTED_EDGE('',*,*,#6858,.T.);
#9290=ORIENTED_EDGE('',*,*,#6900,.F.);
#9291=ORIENTED_EDGE('',*,*,#6899,.T.);
#9292=ORIENTED_EDGE('',*,*,#6814,.T.);
#9293=ORIENTED_EDGE('',*,*,#6901,.F.);
#9294=ORIENTED_EDGE('',*,*,#6859,.F.);
#9295=ORIENTED_EDGE('',*,*,#6902,.F.);
#9296=ORIENTED_EDGE('',*,*,#6816,.F.);
#9297=ORIENTED_EDGE('',*,*,#6902,.T.);
#9298=ORIENTED_EDGE('',*,*,#6898,.F.);
#9299=ORIENTED_EDGE('',*,*,#6903,.T.);
#9300=ORIENTED_EDGE('',*,*,#6817,.T.);
#9301=ORIENTED_EDGE('',*,*,#6903,.F.);
#9302=ORIENTED_EDGE('',*,*,#6897,.F.);
#9303=ORIENTED_EDGE('',*,*,#6904,.F.);
#9304=ORIENTED_EDGE('',*,*,#6818,.F.);
#9305=ORIENTED_EDGE('',*,*,#6904,.T.);
#9306=ORIENTED_EDGE('',*,*,#6896,.F.);
#9307=ORIENTED_EDGE('',*,*,#6905,.T.);
#9308=ORIENTED_EDGE('',*,*,#6819,.T.);
#9309=ORIENTED_EDGE('',*,*,#6905,.F.);
#9310=ORIENTED_EDGE('',*,*,#6895,.F.);
#9311=ORIENTED_EDGE('',*,*,#6906,.F.);
#9312=ORIENTED_EDGE('',*,*,#6820,.F.);
#9313=ORIENTED_EDGE('',*,*,#6906,.T.);
#9314=ORIENTED_EDGE('',*,*,#6894,.F.);
#9315=ORIENTED_EDGE('',*,*,#6907,.T.);
#9316=ORIENTED_EDGE('',*,*,#6821,.T.);
#9317=ORIENTED_EDGE('',*,*,#6907,.F.);
#9318=ORIENTED_EDGE('',*,*,#6893,.F.);
#9319=ORIENTED_EDGE('',*,*,#6908,.F.);
#9320=ORIENTED_EDGE('',*,*,#6822,.F.);
#9321=ORIENTED_EDGE('',*,*,#6908,.T.);
#9322=ORIENTED_EDGE('',*,*,#6892,.F.);
#9323=ORIENTED_EDGE('',*,*,#6909,.T.);
#9324=ORIENTED_EDGE('',*,*,#6823,.T.);
#9325=ORIENTED_EDGE('',*,*,#6909,.F.);
#9326=ORIENTED_EDGE('',*,*,#6891,.F.);
#9327=ORIENTED_EDGE('',*,*,#6910,.F.);
#9328=ORIENTED_EDGE('',*,*,#6824,.F.);
#9329=ORIENTED_EDGE('',*,*,#6910,.T.);
#9330=ORIENTED_EDGE('',*,*,#6890,.F.);
#9331=ORIENTED_EDGE('',*,*,#6911,.T.);
#9332=ORIENTED_EDGE('',*,*,#6825,.T.);
#9333=ORIENTED_EDGE('',*,*,#6911,.F.);
#9334=ORIENTED_EDGE('',*,*,#6889,.F.);
#9335=ORIENTED_EDGE('',*,*,#6912,.F.);
#9336=ORIENTED_EDGE('',*,*,#6826,.F.);
#9337=ORIENTED_EDGE('',*,*,#6912,.T.);
#9338=ORIENTED_EDGE('',*,*,#6888,.F.);
#9339=ORIENTED_EDGE('',*,*,#6913,.T.);
#9340=ORIENTED_EDGE('',*,*,#6827,.T.);
#9341=ORIENTED_EDGE('',*,*,#6913,.F.);
#9342=ORIENTED_EDGE('',*,*,#6887,.F.);
#9343=ORIENTED_EDGE('',*,*,#6914,.F.);
#9344=ORIENTED_EDGE('',*,*,#6828,.F.);
#9345=ORIENTED_EDGE('',*,*,#6914,.T.);
#9346=ORIENTED_EDGE('',*,*,#6886,.F.);
#9347=ORIENTED_EDGE('',*,*,#6915,.T.);
#9348=ORIENTED_EDGE('',*,*,#6829,.T.);
#9349=ORIENTED_EDGE('',*,*,#6915,.F.);
#9350=ORIENTED_EDGE('',*,*,#6885,.F.);
#9351=ORIENTED_EDGE('',*,*,#6916,.F.);
#9352=ORIENTED_EDGE('',*,*,#6830,.F.);
#9353=ORIENTED_EDGE('',*,*,#6916,.T.);
#9354=ORIENTED_EDGE('',*,*,#6884,.F.);
#9355=ORIENTED_EDGE('',*,*,#6917,.T.);
#9356=ORIENTED_EDGE('',*,*,#6831,.T.);
#9357=ORIENTED_EDGE('',*,*,#6917,.F.);
#9358=ORIENTED_EDGE('',*,*,#6883,.F.);
#9359=ORIENTED_EDGE('',*,*,#6918,.F.);
#9360=ORIENTED_EDGE('',*,*,#6832,.F.);
#9361=ORIENTED_EDGE('',*,*,#6918,.T.);
#9362=ORIENTED_EDGE('',*,*,#6882,.F.);
#9363=ORIENTED_EDGE('',*,*,#6919,.T.);
#9364=ORIENTED_EDGE('',*,*,#6833,.T.);
#9365=ORIENTED_EDGE('',*,*,#6919,.F.);
#9366=ORIENTED_EDGE('',*,*,#6881,.F.);
#9367=ORIENTED_EDGE('',*,*,#6920,.F.);
#9368=ORIENTED_EDGE('',*,*,#6834,.F.);
#9369=ORIENTED_EDGE('',*,*,#6920,.T.);
#9370=ORIENTED_EDGE('',*,*,#6880,.F.);
#9371=ORIENTED_EDGE('',*,*,#6921,.T.);
#9372=ORIENTED_EDGE('',*,*,#6835,.T.);
#9373=ORIENTED_EDGE('',*,*,#6921,.F.);
#9374=ORIENTED_EDGE('',*,*,#6879,.F.);
#9375=ORIENTED_EDGE('',*,*,#6922,.F.);
#9376=ORIENTED_EDGE('',*,*,#6836,.F.);
#9377=ORIENTED_EDGE('',*,*,#6922,.T.);
#9378=ORIENTED_EDGE('',*,*,#6878,.F.);
#9379=ORIENTED_EDGE('',*,*,#6923,.T.);
#9380=ORIENTED_EDGE('',*,*,#6837,.T.);
#9381=ORIENTED_EDGE('',*,*,#6923,.F.);
#9382=ORIENTED_EDGE('',*,*,#6877,.F.);
#9383=ORIENTED_EDGE('',*,*,#6924,.F.);
#9384=ORIENTED_EDGE('',*,*,#6838,.F.);
#9385=ORIENTED_EDGE('',*,*,#6924,.T.);
#9386=ORIENTED_EDGE('',*,*,#6876,.F.);
#9387=ORIENTED_EDGE('',*,*,#6925,.T.);
#9388=ORIENTED_EDGE('',*,*,#6839,.T.);
#9389=ORIENTED_EDGE('',*,*,#6925,.F.);
#9390=ORIENTED_EDGE('',*,*,#6875,.F.);
#9391=ORIENTED_EDGE('',*,*,#6926,.F.);
#9392=ORIENTED_EDGE('',*,*,#6840,.F.);
#9393=ORIENTED_EDGE('',*,*,#6926,.T.);
#9394=ORIENTED_EDGE('',*,*,#6874,.F.);
#9395=ORIENTED_EDGE('',*,*,#6927,.T.);
#9396=ORIENTED_EDGE('',*,*,#6841,.T.);
#9397=ORIENTED_EDGE('',*,*,#6927,.F.);
#9398=ORIENTED_EDGE('',*,*,#6873,.F.);
#9399=ORIENTED_EDGE('',*,*,#6928,.F.);
#9400=ORIENTED_EDGE('',*,*,#6842,.F.);
#9401=ORIENTED_EDGE('',*,*,#6928,.T.);
#9402=ORIENTED_EDGE('',*,*,#6872,.F.);
#9403=ORIENTED_EDGE('',*,*,#6929,.T.);
#9404=ORIENTED_EDGE('',*,*,#6843,.T.);
#9405=ORIENTED_EDGE('',*,*,#6929,.F.);
#9406=ORIENTED_EDGE('',*,*,#6871,.F.);
#9407=ORIENTED_EDGE('',*,*,#6930,.F.);
#9408=ORIENTED_EDGE('',*,*,#6844,.F.);
#9409=ORIENTED_EDGE('',*,*,#6930,.T.);
#9410=ORIENTED_EDGE('',*,*,#6870,.F.);
#9411=ORIENTED_EDGE('',*,*,#6931,.T.);
#9412=ORIENTED_EDGE('',*,*,#6845,.T.);
#9413=ORIENTED_EDGE('',*,*,#6931,.F.);
#9414=ORIENTED_EDGE('',*,*,#6869,.F.);
#9415=ORIENTED_EDGE('',*,*,#6932,.F.);
#9416=ORIENTED_EDGE('',*,*,#6846,.F.);
#9417=ORIENTED_EDGE('',*,*,#6932,.T.);
#9418=ORIENTED_EDGE('',*,*,#6868,.F.);
#9419=ORIENTED_EDGE('',*,*,#6933,.T.);
#9420=ORIENTED_EDGE('',*,*,#6847,.T.);
#9421=ORIENTED_EDGE('',*,*,#6933,.F.);
#9422=ORIENTED_EDGE('',*,*,#6867,.F.);
#9423=ORIENTED_EDGE('',*,*,#6934,.F.);
#9424=ORIENTED_EDGE('',*,*,#6848,.F.);
#9425=ORIENTED_EDGE('',*,*,#6934,.T.);
#9426=ORIENTED_EDGE('',*,*,#6866,.F.);
#9427=ORIENTED_EDGE('',*,*,#6935,.T.);
#9428=ORIENTED_EDGE('',*,*,#6849,.T.);
#9429=ORIENTED_EDGE('',*,*,#6935,.F.);
#9430=ORIENTED_EDGE('',*,*,#6865,.F.);
#9431=ORIENTED_EDGE('',*,*,#6936,.F.);
#9432=ORIENTED_EDGE('',*,*,#6850,.F.);
#9433=ORIENTED_EDGE('',*,*,#6936,.T.);
#9434=ORIENTED_EDGE('',*,*,#6864,.F.);
#9435=ORIENTED_EDGE('',*,*,#6937,.T.);
#9436=ORIENTED_EDGE('',*,*,#6851,.T.);
#9437=ORIENTED_EDGE('',*,*,#6938,.F.);
#9438=ORIENTED_EDGE('',*,*,#6852,.F.);
#9439=ORIENTED_EDGE('',*,*,#6937,.F.);
#9440=ORIENTED_EDGE('',*,*,#6863,.F.);
#9441=ORIENTED_EDGE('',*,*,#6901,.T.);
#9442=ORIENTED_EDGE('',*,*,#6855,.T.);
#9443=ORIENTED_EDGE('',*,*,#6939,.T.);
#9444=ORIENTED_EDGE('',*,*,#6860,.F.);
#9445=ORIENTED_EDGE('',*,*,#6940,.F.);
#9446=ORIENTED_EDGE('',*,*,#6861,.F.);
#9447=ORIENTED_EDGE('',*,*,#6939,.F.);
#9448=ORIENTED_EDGE('',*,*,#6854,.F.);
#9449=ORIENTED_EDGE('',*,*,#6938,.T.);
#9450=ORIENTED_EDGE('',*,*,#6862,.F.);
#9451=ORIENTED_EDGE('',*,*,#6940,.T.);
#9452=ORIENTED_EDGE('',*,*,#6853,.T.);
#10227=CYLINDRICAL_SURFACE('',#12321,0.125);
#10228=CYLINDRICAL_SURFACE('',#12322,0.125);
#10229=CYLINDRICAL_SURFACE('',#12323,0.65);
#10230=CYLINDRICAL_SURFACE('',#12326,0.125);
#10231=CYLINDRICAL_SURFACE('',#12327,0.125);
#10232=CYLINDRICAL_SURFACE('',#12328,0.4);
#10233=CYLINDRICAL_SURFACE('',#12374,0.8);
#10234=CYLINDRICAL_SURFACE('',#12419,0.8);
#10235=CYLINDRICAL_SURFACE('',#12422,0.0555);
#10236=CYLINDRICAL_SURFACE('',#12423,0.611219772367581);
#10237=CYLINDRICAL_SURFACE('',#12424,0.0555);
#10238=CYLINDRICAL_SURFACE('',#12425,0.611219772367581);
#10239=CYLINDRICAL_SURFACE('',#12426,0.0555);
#10240=CYLINDRICAL_SURFACE('',#12427,0.611219772367581);
#10241=CYLINDRICAL_SURFACE('',#12428,0.0555);
#10242=CYLINDRICAL_SURFACE('',#12429,0.611219772367581);
#10243=CYLINDRICAL_SURFACE('',#12430,0.0555);
#10244=CYLINDRICAL_SURFACE('',#12431,0.611219772367581);
#10245=CYLINDRICAL_SURFACE('',#12432,0.0555);
#10246=CYLINDRICAL_SURFACE('',#12433,0.611219772367581);
#10247=CYLINDRICAL_SURFACE('',#12434,0.0555);
#10248=CYLINDRICAL_SURFACE('',#12435,0.611219772367581);
#10249=CYLINDRICAL_SURFACE('',#12436,0.0555);
#10250=CYLINDRICAL_SURFACE('',#12437,0.611219772367581);
#10251=CYLINDRICAL_SURFACE('',#12438,0.0555);
#10252=CYLINDRICAL_SURFACE('',#12439,0.611219772367581);
#10253=CYLINDRICAL_SURFACE('',#12440,0.0555);
#10254=CYLINDRICAL_SURFACE('',#12441,0.611219772367581);
#10255=CYLINDRICAL_SURFACE('',#12442,0.0555);
#10256=CYLINDRICAL_SURFACE('',#12443,0.611219772367581);
#10257=CYLINDRICAL_SURFACE('',#12444,0.0555);
#10258=CYLINDRICAL_SURFACE('',#12445,0.611219772367581);
#10259=CYLINDRICAL_SURFACE('',#12446,0.0555);
#10260=CYLINDRICAL_SURFACE('',#12447,0.611219772367581);
#10261=CYLINDRICAL_SURFACE('',#12448,0.0555);
#10262=CYLINDRICAL_SURFACE('',#12449,0.611219772367581);
#10263=CYLINDRICAL_SURFACE('',#12450,0.0555);
#10264=CYLINDRICAL_SURFACE('',#12451,0.611219772367581);
#10265=CYLINDRICAL_SURFACE('',#12452,0.0555);
#10266=CYLINDRICAL_SURFACE('',#12453,0.611219772367581);
#10267=CYLINDRICAL_SURFACE('',#12454,0.0555);
#10268=CYLINDRICAL_SURFACE('',#12455,0.611219772367581);
#10269=CYLINDRICAL_SURFACE('',#12456,0.0555);
#10270=CYLINDRICAL_SURFACE('',#12457,0.611219772367581);
#10271=CYLINDRICAL_SURFACE('',#12458,0.0555);
#10272=CYLINDRICAL_SURFACE('',#12459,0.611219772367581);
#10273=CYLINDRICAL_SURFACE('',#12460,0.0555);
#10274=CYLINDRICAL_SURFACE('',#12461,0.611219772367581);
#10731=ADVANCED_FACE('',(#1680),#10227,.F.);
#10732=ADVANCED_FACE('',(#1681),#10228,.F.);
#10733=ADVANCED_FACE('',(#1682,#851,#852,#853),#10229,.T.);
#10734=ADVANCED_FACE('',(#1683),#10230,.F.);
#10735=ADVANCED_FACE('',(#1684),#10231,.F.);
#10736=ADVANCED_FACE('',(#1685,#854,#855,#856),#10232,.F.);
#10737=ADVANCED_FACE('',(#1686,#857),#1144,.F.);
#10738=ADVANCED_FACE('',(#1687,#858),#1145,.T.);
#10739=ADVANCED_FACE('',(#1688),#10233,.T.);
#10740=ADVANCED_FACE('',(#1689,#859),#1146,.F.);
#10741=ADVANCED_FACE('',(#1690,#860),#1147,.F.);
#10742=ADVANCED_FACE('',(#1691),#10234,.T.);
#10743=ADVANCED_FACE('',(#1692,#861),#1148,.T.);
#10744=ADVANCED_FACE('',(#1693),#10235,.F.);
#10745=ADVANCED_FACE('',(#1694),#10236,.T.);
#10746=ADVANCED_FACE('',(#1695),#10237,.F.);
#10747=ADVANCED_FACE('',(#1696),#10238,.T.);
#10748=ADVANCED_FACE('',(#1697),#10239,.F.);
#10749=ADVANCED_FACE('',(#1698),#10240,.T.);
#10750=ADVANCED_FACE('',(#1699),#10241,.F.);
#10751=ADVANCED_FACE('',(#1700),#10242,.T.);
#10752=ADVANCED_FACE('',(#1701),#10243,.F.);
#10753=ADVANCED_FACE('',(#1702),#10244,.T.);
#10754=ADVANCED_FACE('',(#1703),#10245,.F.);
#10755=ADVANCED_FACE('',(#1704),#10246,.T.);
#10756=ADVANCED_FACE('',(#1705),#10247,.F.);
#10757=ADVANCED_FACE('',(#1706),#10248,.T.);
#10758=ADVANCED_FACE('',(#1707),#10249,.F.);
#10759=ADVANCED_FACE('',(#1708),#10250,.T.);
#10760=ADVANCED_FACE('',(#1709),#10251,.F.);
#10761=ADVANCED_FACE('',(#1710),#10252,.T.);
#10762=ADVANCED_FACE('',(#1711),#10253,.F.);
#10763=ADVANCED_FACE('',(#1712),#10254,.T.);
#10764=ADVANCED_FACE('',(#1713),#10255,.F.);
#10765=ADVANCED_FACE('',(#1714),#10256,.T.);
#10766=ADVANCED_FACE('',(#1715),#10257,.F.);
#10767=ADVANCED_FACE('',(#1716),#10258,.T.);
#10768=ADVANCED_FACE('',(#1717),#10259,.F.);
#10769=ADVANCED_FACE('',(#1718),#10260,.T.);
#10770=ADVANCED_FACE('',(#1719),#10261,.F.);
#10771=ADVANCED_FACE('',(#1720),#10262,.T.);
#10772=ADVANCED_FACE('',(#1721),#10263,.F.);
#10773=ADVANCED_FACE('',(#1722),#10264,.T.);
#10774=ADVANCED_FACE('',(#1723),#10265,.F.);
#10775=ADVANCED_FACE('',(#1724),#10266,.T.);
#10776=ADVANCED_FACE('',(#1725),#10267,.F.);
#10777=ADVANCED_FACE('',(#1726),#10268,.T.);
#10778=ADVANCED_FACE('',(#1727),#10269,.F.);
#10779=ADVANCED_FACE('',(#1728),#10270,.T.);
#10780=ADVANCED_FACE('',(#1729),#10271,.F.);
#10781=ADVANCED_FACE('',(#1730),#10272,.T.);
#10782=ADVANCED_FACE('',(#1731),#10273,.F.);
#10783=ADVANCED_FACE('',(#1732),#10274,.T.);
#10969=CLOSED_SHELL('',(#10731,#10732,#10733,#10734,#10735,#10736,#10737,
#10738,#10739,#10740,#10741,#10742,#10743,#10744,#10745,#10746,#10747,#10748,
#10749,#10750,#10751,#10752,#10753,#10754,#10755,#10756,#10757,#10758,#10759,
#10760,#10761,#10762,#10763,#10764,#10765,#10766,#10767,#10768,#10769,#10770,
#10771,#10772,#10773,#10774,#10775,#10776,#10777,#10778,#10779,#10780,#10781,
#10782,#10783));
#12320=AXIS2_PLACEMENT_3D('',#18620,#15012,#15013);
#12321=AXIS2_PLACEMENT_3D('',#18621,#15014,#15015);
#12322=AXIS2_PLACEMENT_3D('',#18708,#15017,#15018);
#12323=AXIS2_PLACEMENT_3D('',#18789,#15020,#15021);
#12324=AXIS2_PLACEMENT_3D('',#18791,#15022,#15023);
#12325=AXIS2_PLACEMENT_3D('',#18795,#15026,#15027);
#12326=AXIS2_PLACEMENT_3D('',#18878,#15028,#15029);
#12327=AXIS2_PLACEMENT_3D('',#18918,#15031,#15032);
#12328=AXIS2_PLACEMENT_3D('',#18958,#15034,#15035);
#12329=AXIS2_PLACEMENT_3D('',#18960,#15036,#15037);
#12330=AXIS2_PLACEMENT_3D('',#18964,#15040,#15041);
#12331=AXIS2_PLACEMENT_3D('',#18965,#15042,#15043);
#12332=AXIS2_PLACEMENT_3D('',#18966,#15044,#15045);
#12333=AXIS2_PLACEMENT_3D('',#18968,#15046,#15047);
#12334=AXIS2_PLACEMENT_3D('',#18971,#15048,#15049);
#12335=AXIS2_PLACEMENT_3D('',#18973,#15050,#15051);
#12336=AXIS2_PLACEMENT_3D('',#18975,#15052,#15053);
#12337=AXIS2_PLACEMENT_3D('',#18977,#15054,#15055);
#12338=AXIS2_PLACEMENT_3D('',#18979,#15056,#15057);
#12339=AXIS2_PLACEMENT_3D('',#18981,#15058,#15059);
#12340=AXIS2_PLACEMENT_3D('',#18983,#15060,#15061);
#12341=AXIS2_PLACEMENT_3D('',#18985,#15062,#15063);
#12342=AXIS2_PLACEMENT_3D('',#18987,#15064,#15065);
#12343=AXIS2_PLACEMENT_3D('',#18989,#15066,#15067);
#12344=AXIS2_PLACEMENT_3D('',#18991,#15068,#15069);
#12345=AXIS2_PLACEMENT_3D('',#18993,#15070,#15071);
#12346=AXIS2_PLACEMENT_3D('',#18995,#15072,#15073);
#12347=AXIS2_PLACEMENT_3D('',#18997,#15074,#15075);
#12348=AXIS2_PLACEMENT_3D('',#18999,#15076,#15077);
#12349=AXIS2_PLACEMENT_3D('',#19001,#15078,#15079);
#12350=AXIS2_PLACEMENT_3D('',#19003,#15080,#15081);
#12351=AXIS2_PLACEMENT_3D('',#19005,#15082,#15083);
#12352=AXIS2_PLACEMENT_3D('',#19007,#15084,#15085);
#12353=AXIS2_PLACEMENT_3D('',#19009,#15086,#15087);
#12354=AXIS2_PLACEMENT_3D('',#19011,#15088,#15089);
#12355=AXIS2_PLACEMENT_3D('',#19013,#15090,#15091);
#12356=AXIS2_PLACEMENT_3D('',#19015,#15092,#15093);
#12357=AXIS2_PLACEMENT_3D('',#19017,#15094,#15095);
#12358=AXIS2_PLACEMENT_3D('',#19019,#15096,#15097);
#12359=AXIS2_PLACEMENT_3D('',#19021,#15098,#15099);
#12360=AXIS2_PLACEMENT_3D('',#19023,#15100,#15101);
#12361=AXIS2_PLACEMENT_3D('',#19025,#15102,#15103);
#12362=AXIS2_PLACEMENT_3D('',#19027,#15104,#15105);
#12363=AXIS2_PLACEMENT_3D('',#19029,#15106,#15107);
#12364=AXIS2_PLACEMENT_3D('',#19031,#15108,#15109);
#12365=AXIS2_PLACEMENT_3D('',#19033,#15110,#15111);
#12366=AXIS2_PLACEMENT_3D('',#19035,#15112,#15113);
#12367=AXIS2_PLACEMENT_3D('',#19037,#15114,#15115);
#12368=AXIS2_PLACEMENT_3D('',#19039,#15116,#15117);
#12369=AXIS2_PLACEMENT_3D('',#19041,#15118,#15119);
#12370=AXIS2_PLACEMENT_3D('',#19043,#15120,#15121);
#12371=AXIS2_PLACEMENT_3D('',#19045,#15122,#15123);
#12372=AXIS2_PLACEMENT_3D('',#19047,#15124,#15125);
#12373=AXIS2_PLACEMENT_3D('',#19048,#15126,#15127);
#12374=AXIS2_PLACEMENT_3D('',#19049,#15128,#15129);
#12375=AXIS2_PLACEMENT_3D('',#19051,#15130,#15131);
#12376=AXIS2_PLACEMENT_3D('',#19053,#15133,#15134);
#12377=AXIS2_PLACEMENT_3D('',#19054,#15135,#15136);
#12378=AXIS2_PLACEMENT_3D('',#19056,#15137,#15138);
#12379=AXIS2_PLACEMENT_3D('',#19059,#15139,#15140);
#12380=AXIS2_PLACEMENT_3D('',#19061,#15141,#15142);
#12381=AXIS2_PLACEMENT_3D('',#19063,#15143,#15144);
#12382=AXIS2_PLACEMENT_3D('',#19065,#15145,#15146);
#12383=AXIS2_PLACEMENT_3D('',#19067,#15147,#15148);
#12384=AXIS2_PLACEMENT_3D('',#19069,#15149,#15150);
#12385=AXIS2_PLACEMENT_3D('',#19071,#15151,#15152);
#12386=AXIS2_PLACEMENT_3D('',#19073,#15153,#15154);
#12387=AXIS2_PLACEMENT_3D('',#19075,#15155,#15156);
#12388=AXIS2_PLACEMENT_3D('',#19077,#15157,#15158);
#12389=AXIS2_PLACEMENT_3D('',#19079,#15159,#15160);
#12390=AXIS2_PLACEMENT_3D('',#19081,#15161,#15162);
#12391=AXIS2_PLACEMENT_3D('',#19083,#15163,#15164);
#12392=AXIS2_PLACEMENT_3D('',#19085,#15165,#15166);
#12393=AXIS2_PLACEMENT_3D('',#19087,#15167,#15168);
#12394=AXIS2_PLACEMENT_3D('',#19089,#15169,#15170);
#12395=AXIS2_PLACEMENT_3D('',#19091,#15171,#15172);
#12396=AXIS2_PLACEMENT_3D('',#19093,#15173,#15174);
#12397=AXIS2_PLACEMENT_3D('',#19095,#15175,#15176);
#12398=AXIS2_PLACEMENT_3D('',#19097,#15177,#15178);
#12399=AXIS2_PLACEMENT_3D('',#19099,#15179,#15180);
#12400=AXIS2_PLACEMENT_3D('',#19101,#15181,#15182);
#12401=AXIS2_PLACEMENT_3D('',#19103,#15183,#15184);
#12402=AXIS2_PLACEMENT_3D('',#19105,#15185,#15186);
#12403=AXIS2_PLACEMENT_3D('',#19107,#15187,#15188);
#12404=AXIS2_PLACEMENT_3D('',#19109,#15189,#15190);
#12405=AXIS2_PLACEMENT_3D('',#19111,#15191,#15192);
#12406=AXIS2_PLACEMENT_3D('',#19113,#15193,#15194);
#12407=AXIS2_PLACEMENT_3D('',#19115,#15195,#15196);
#12408=AXIS2_PLACEMENT_3D('',#19117,#15197,#15198);
#12409=AXIS2_PLACEMENT_3D('',#19119,#15199,#15200);
#12410=AXIS2_PLACEMENT_3D('',#19121,#15201,#15202);
#12411=AXIS2_PLACEMENT_3D('',#19123,#15203,#15204);
#12412=AXIS2_PLACEMENT_3D('',#19125,#15205,#15206);
#12413=AXIS2_PLACEMENT_3D('',#19127,#15207,#15208);
#12414=AXIS2_PLACEMENT_3D('',#19129,#15209,#15210);
#12415=AXIS2_PLACEMENT_3D('',#19131,#15211,#15212);
#12416=AXIS2_PLACEMENT_3D('',#19133,#15213,#15214);
#12417=AXIS2_PLACEMENT_3D('',#19135,#15215,#15216);
#12418=AXIS2_PLACEMENT_3D('',#19136,#15217,#15218);
#12419=AXIS2_PLACEMENT_3D('',#19137,#15219,#15220);
#12420=AXIS2_PLACEMENT_3D('',#19139,#15221,#15222);
#12421=AXIS2_PLACEMENT_3D('',#19141,#15224,#15225);
#12422=AXIS2_PLACEMENT_3D('',#19142,#15226,#15227);
#12423=AXIS2_PLACEMENT_3D('',#19145,#15230,#15231);
#12424=AXIS2_PLACEMENT_3D('',#19147,#15233,#15234);
#12425=AXIS2_PLACEMENT_3D('',#19149,#15236,#15237);
#12426=AXIS2_PLACEMENT_3D('',#19151,#15239,#15240);
#12427=AXIS2_PLACEMENT_3D('',#19153,#15242,#15243);
#12428=AXIS2_PLACEMENT_3D('',#19155,#15245,#15246);
#12429=AXIS2_PLACEMENT_3D('',#19157,#15248,#15249);
#12430=AXIS2_PLACEMENT_3D('',#19159,#15251,#15252);
#12431=AXIS2_PLACEMENT_3D('',#19161,#15254,#15255);
#12432=AXIS2_PLACEMENT_3D('',#19163,#15257,#15258);
#12433=AXIS2_PLACEMENT_3D('',#19165,#15260,#15261);
#12434=AXIS2_PLACEMENT_3D('',#19167,#15263,#15264);
#12435=AXIS2_PLACEMENT_3D('',#19169,#15266,#15267);
#12436=AXIS2_PLACEMENT_3D('',#19171,#15269,#15270);
#12437=AXIS2_PLACEMENT_3D('',#19173,#15272,#15273);
#12438=AXIS2_PLACEMENT_3D('',#19175,#15275,#15276);
#12439=AXIS2_PLACEMENT_3D('',#19177,#15278,#15279);
#12440=AXIS2_PLACEMENT_3D('',#19179,#15281,#15282);
#12441=AXIS2_PLACEMENT_3D('',#19181,#15284,#15285);
#12442=AXIS2_PLACEMENT_3D('',#19183,#15287,#15288);
#12443=AXIS2_PLACEMENT_3D('',#19185,#15290,#15291);
#12444=AXIS2_PLACEMENT_3D('',#19187,#15293,#15294);
#12445=AXIS2_PLACEMENT_3D('',#19189,#15296,#15297);
#12446=AXIS2_PLACEMENT_3D('',#19191,#15299,#15300);
#12447=AXIS2_PLACEMENT_3D('',#19193,#15302,#15303);
#12448=AXIS2_PLACEMENT_3D('',#19195,#15305,#15306);
#12449=AXIS2_PLACEMENT_3D('',#19197,#15308,#15309);
#12450=AXIS2_PLACEMENT_3D('',#19199,#15311,#15312);
#12451=AXIS2_PLACEMENT_3D('',#19201,#15314,#15315);
#12452=AXIS2_PLACEMENT_3D('',#19203,#15317,#15318);
#12453=AXIS2_PLACEMENT_3D('',#19205,#15320,#15321);
#12454=AXIS2_PLACEMENT_3D('',#19207,#15323,#15324);
#12455=AXIS2_PLACEMENT_3D('',#19209,#15326,#15327);
#12456=AXIS2_PLACEMENT_3D('',#19211,#15329,#15330);
#12457=AXIS2_PLACEMENT_3D('',#19213,#15332,#15333);
#12458=AXIS2_PLACEMENT_3D('',#19215,#15335,#15336);
#12459=AXIS2_PLACEMENT_3D('',#19217,#15338,#15339);
#12460=AXIS2_PLACEMENT_3D('',#19219,#15341,#15342);
#12461=AXIS2_PLACEMENT_3D('',#19221,#15344,#15345);
#15012=DIRECTION('axis',(0.,0.,1.));
#15013=DIRECTION('refdir',(1.,0.,0.));
#15014=DIRECTION('center_axis',(1.,0.,6.12323399573677E-17));
#15015=DIRECTION('ref_axis',(6.12323399573677E-17,0.,-1.));
#15016=DIRECTION('',(1.,0.,6.12323399573677E-17));
#15017=DIRECTION('center_axis',(1.,0.,6.12323399573677E-17));
#15018=DIRECTION('ref_axis',(6.12323399573677E-17,0.,-1.));
#15019=DIRECTION('',(1.,0.,6.12323399573677E-17));
#15020=DIRECTION('center_axis',(0.,-1.,0.));
#15021=DIRECTION('ref_axis',(1.,0.,0.));
#15022=DIRECTION('center_axis',(0.,-1.,0.));
#15023=DIRECTION('ref_axis',(1.,0.,0.));
#15024=DIRECTION('',(0.,1.,0.));
#15025=DIRECTION('',(0.,1.,0.));
#15026=DIRECTION('center_axis',(0.,1.,0.));
#15027=DIRECTION('ref_axis',(1.,0.,0.));
#15028=DIRECTION('center_axis',(0.,0.,1.));
#15029=DIRECTION('ref_axis',(1.,0.,0.));
#15030=DIRECTION('',(0.,0.,1.));
#15031=DIRECTION('center_axis',(0.,0.,1.));
#15032=DIRECTION('ref_axis',(1.,0.,0.));
#15033=DIRECTION('',(0.,0.,1.));
#15034=DIRECTION('center_axis',(0.,1.,0.));
#15035=DIRECTION('ref_axis',(1.,0.,0.));
#15036=DIRECTION('center_axis',(0.,1.,0.));
#15037=DIRECTION('ref_axis',(1.,0.,0.));
#15038=DIRECTION('',(0.,1.,0.));
#15039=DIRECTION('',(0.,1.,0.));
#15040=DIRECTION('center_axis',(0.,-1.,0.));
#15041=DIRECTION('ref_axis',(1.,0.,0.));
#15042=DIRECTION('center_axis',(0.,1.,0.));
#15043=DIRECTION('ref_axis',(1.,0.,0.));
#15044=DIRECTION('center_axis',(0.,1.,0.));
#15045=DIRECTION('ref_axis',(1.,0.,0.));
#15046=DIRECTION('center_axis',(0.,1.,0.));
#15047=DIRECTION('ref_axis',(1.,0.,0.));
#15048=DIRECTION('center_axis',(0.,1.,0.));
#15049=DIRECTION('ref_axis',(0.951056516295154,0.,0.309016994374948));
#15050=DIRECTION('center_axis',(0.,1.,0.));
#15051=DIRECTION('ref_axis',(1.,0.,0.));
#15052=DIRECTION('center_axis',(0.,1.,0.));
#15053=DIRECTION('ref_axis',(0.809016994374947,0.,0.587785252292473));
#15054=DIRECTION('center_axis',(0.,1.,0.));
#15055=DIRECTION('ref_axis',(1.,0.,0.));
#15056=DIRECTION('center_axis',(0.,1.,0.));
#15057=DIRECTION('ref_axis',(0.587785252292473,0.,0.809016994374948));
#15058=DIRECTION('center_axis',(0.,1.,0.));
#15059=DIRECTION('ref_axis',(1.,0.,0.));
#15060=DIRECTION('center_axis',(0.,1.,0.));
#15061=DIRECTION('ref_axis',(0.309016994374947,0.,0.951056516295154));
#15062=DIRECTION('center_axis',(0.,1.,0.));
#15063=DIRECTION('ref_axis',(1.,0.,0.));
#15064=DIRECTION('center_axis',(0.,1.,0.));
#15065=DIRECTION('ref_axis',(-1.83697019872103E-16,0.,1.));
#15066=DIRECTION('center_axis',(0.,1.,0.));
#15067=DIRECTION('ref_axis',(1.,0.,0.));
#15068=DIRECTION('center_axis',(0.,1.,0.));
#15069=DIRECTION('ref_axis',(-0.309016994374948,0.,0.951056516295154));
#15070=DIRECTION('center_axis',(0.,1.,0.));
#15071=DIRECTION('ref_axis',(1.,0.,0.));
#15072=DIRECTION('center_axis',(0.,1.,0.));
#15073=DIRECTION('ref_axis',(-0.587785252292473,0.,0.809016994374947));
#15074=DIRECTION('center_axis',(0.,1.,0.));
#15075=DIRECTION('ref_axis',(1.,0.,0.));
#15076=DIRECTION('center_axis',(0.,1.,0.));
#15077=DIRECTION('ref_axis',(-0.809016994374947,0.,0.587785252292473));
#15078=DIRECTION('center_axis',(0.,1.,0.));
#15079=DIRECTION('ref_axis',(1.,0.,0.));
#15080=DIRECTION('center_axis',(0.,1.,0.));
#15081=DIRECTION('ref_axis',(-0.951056516295154,0.,0.309016994374947));
#15082=DIRECTION('center_axis',(0.,1.,0.));
#15083=DIRECTION('ref_axis',(1.,0.,0.));
#15084=DIRECTION('center_axis',(0.,1.,0.));
#15085=DIRECTION('ref_axis',(-1.,0.,-1.22464679914735E-16));
#15086=DIRECTION('center_axis',(0.,1.,0.));
#15087=DIRECTION('ref_axis',(1.,0.,0.));
#15088=DIRECTION('center_axis',(0.,1.,0.));
#15089=DIRECTION('ref_axis',(-0.951056516295154,0.,-0.309016994374948));
#15090=DIRECTION('center_axis',(0.,1.,0.));
#15091=DIRECTION('ref_axis',(1.,0.,0.));
#15092=DIRECTION('center_axis',(0.,1.,0.));
#15093=DIRECTION('ref_axis',(-0.809016994374947,0.,-0.587785252292473));
#15094=DIRECTION('center_axis',(0.,1.,0.));
#15095=DIRECTION('ref_axis',(1.,0.,0.));
#15096=DIRECTION('center_axis',(0.,1.,0.));
#15097=DIRECTION('ref_axis',(-0.587785252292473,0.,-0.809016994374948));
#15098=DIRECTION('center_axis',(0.,1.,0.));
#15099=DIRECTION('ref_axis',(1.,0.,0.));
#15100=DIRECTION('center_axis',(0.,1.,0.));
#15101=DIRECTION('ref_axis',(-0.309016994374947,0.,-0.951056516295154));
#15102=DIRECTION('center_axis',(0.,1.,0.));
#15103=DIRECTION('ref_axis',(1.,0.,0.));
#15104=DIRECTION('center_axis',(0.,1.,0.));
#15105=DIRECTION('ref_axis',(6.12323399573677E-17,0.,-1.));
#15106=DIRECTION('center_axis',(0.,1.,0.));
#15107=DIRECTION('ref_axis',(1.,0.,0.));
#15108=DIRECTION('center_axis',(0.,1.,0.));
#15109=DIRECTION('ref_axis',(0.309016994374947,0.,-0.951056516295154));
#15110=DIRECTION('center_axis',(0.,1.,0.));
#15111=DIRECTION('ref_axis',(1.,0.,0.));
#15112=DIRECTION('center_axis',(0.,1.,0.));
#15113=DIRECTION('ref_axis',(0.587785252292473,0.,-0.809016994374947));
#15114=DIRECTION('center_axis',(0.,1.,0.));
#15115=DIRECTION('ref_axis',(1.,0.,0.));
#15116=DIRECTION('center_axis',(0.,1.,0.));
#15117=DIRECTION('ref_axis',(0.809016994374947,0.,-0.587785252292473));
#15118=DIRECTION('center_axis',(0.,1.,0.));
#15119=DIRECTION('ref_axis',(1.,0.,0.));
#15120=DIRECTION('center_axis',(0.,1.,0.));
#15121=DIRECTION('ref_axis',(0.951056516295154,0.,-0.309016994374947));
#15122=DIRECTION('center_axis',(0.,1.,0.));
#15123=DIRECTION('ref_axis',(1.,0.,0.));
#15124=DIRECTION('center_axis',(0.,1.,0.));
#15125=DIRECTION('ref_axis',(1.,0.,0.));
#15126=DIRECTION('center_axis',(0.,1.,0.));
#15127=DIRECTION('ref_axis',(1.,0.,0.));
#15128=DIRECTION('center_axis',(0.,-1.,0.));
#15129=DIRECTION('ref_axis',(1.,0.,0.));
#15130=DIRECTION('center_axis',(0.,-1.,0.));
#15131=DIRECTION('ref_axis',(1.,0.,0.));
#15132=DIRECTION('',(0.,1.,0.));
#15133=DIRECTION('center_axis',(0.,1.,0.));
#15134=DIRECTION('ref_axis',(1.,0.,0.));
#15135=DIRECTION('center_axis',(0.,1.,0.));
#15136=DIRECTION('ref_axis',(1.,0.,0.));
#15137=DIRECTION('center_axis',(0.,1.,0.));
#15138=DIRECTION('ref_axis',(1.,0.,0.));
#15139=DIRECTION('center_axis',(0.,-1.,0.));
#15140=DIRECTION('ref_axis',(0.951056516295154,0.,0.309016994374948));
#15141=DIRECTION('center_axis',(0.,1.,0.));
#15142=DIRECTION('ref_axis',(1.,0.,0.));
#15143=DIRECTION('center_axis',(0.,-1.,0.));
#15144=DIRECTION('ref_axis',(1.,0.,0.));
#15145=DIRECTION('center_axis',(0.,1.,0.));
#15146=DIRECTION('ref_axis',(1.,0.,0.));
#15147=DIRECTION('center_axis',(0.,-1.,0.));
#15148=DIRECTION('ref_axis',(0.951056516295154,0.,-0.309016994374947));
#15149=DIRECTION('center_axis',(0.,1.,0.));
#15150=DIRECTION('ref_axis',(1.,0.,0.));
#15151=DIRECTION('center_axis',(0.,-1.,0.));
#15152=DIRECTION('ref_axis',(0.809016994374947,0.,-0.587785252292473));
#15153=DIRECTION('center_axis',(0.,1.,0.));
#15154=DIRECTION('ref_axis',(1.,0.,0.));
#15155=DIRECTION('center_axis',(0.,-1.,0.));
#15156=DIRECTION('ref_axis',(0.587785252292473,0.,-0.809016994374947));
#15157=DIRECTION('center_axis',(0.,1.,0.));
#15158=DIRECTION('ref_axis',(1.,0.,0.));
#15159=DIRECTION('center_axis',(0.,-1.,0.));
#15160=DIRECTION('ref_axis',(0.309016994374947,0.,-0.951056516295154));
#15161=DIRECTION('center_axis',(0.,1.,0.));
#15162=DIRECTION('ref_axis',(1.,0.,0.));
#15163=DIRECTION('center_axis',(0.,-1.,0.));
#15164=DIRECTION('ref_axis',(6.12323399573677E-17,0.,-1.));
#15165=DIRECTION('center_axis',(0.,1.,0.));
#15166=DIRECTION('ref_axis',(1.,0.,0.));
#15167=DIRECTION('center_axis',(0.,-1.,0.));
#15168=DIRECTION('ref_axis',(-0.309016994374947,0.,-0.951056516295154));
#15169=DIRECTION('center_axis',(0.,1.,0.));
#15170=DIRECTION('ref_axis',(1.,0.,0.));
#15171=DIRECTION('center_axis',(0.,-1.,0.));
#15172=DIRECTION('ref_axis',(-0.587785252292473,0.,-0.809016994374948));
#15173=DIRECTION('center_axis',(0.,1.,0.));
#15174=DIRECTION('ref_axis',(1.,0.,0.));
#15175=DIRECTION('center_axis',(0.,-1.,0.));
#15176=DIRECTION('ref_axis',(-0.809016994374947,0.,-0.587785252292473));
#15177=DIRECTION('center_axis',(0.,1.,0.));
#15178=DIRECTION('ref_axis',(1.,0.,0.));
#15179=DIRECTION('center_axis',(0.,-1.,0.));
#15180=DIRECTION('ref_axis',(-0.951056516295154,0.,-0.309016994374948));
#15181=DIRECTION('center_axis',(0.,1.,0.));
#15182=DIRECTION('ref_axis',(1.,0.,0.));
#15183=DIRECTION('center_axis',(0.,-1.,0.));
#15184=DIRECTION('ref_axis',(-1.,0.,-1.22464679914735E-16));
#15185=DIRECTION('center_axis',(0.,1.,0.));
#15186=DIRECTION('ref_axis',(1.,0.,0.));
#15187=DIRECTION('center_axis',(0.,-1.,0.));
#15188=DIRECTION('ref_axis',(-0.951056516295154,0.,0.309016994374947));
#15189=DIRECTION('center_axis',(0.,1.,0.));
#15190=DIRECTION('ref_axis',(1.,0.,0.));
#15191=DIRECTION('center_axis',(0.,-1.,0.));
#15192=DIRECTION('ref_axis',(-0.809016994374947,0.,0.587785252292473));
#15193=DIRECTION('center_axis',(0.,1.,0.));
#15194=DIRECTION('ref_axis',(1.,0.,0.));
#15195=DIRECTION('center_axis',(0.,-1.,0.));
#15196=DIRECTION('ref_axis',(-0.587785252292473,0.,0.809016994374947));
#15197=DIRECTION('center_axis',(0.,1.,0.));
#15198=DIRECTION('ref_axis',(1.,0.,0.));
#15199=DIRECTION('center_axis',(0.,-1.,0.));
#15200=DIRECTION('ref_axis',(-0.309016994374948,0.,0.951056516295154));
#15201=DIRECTION('center_axis',(0.,1.,0.));
#15202=DIRECTION('ref_axis',(1.,0.,0.));
#15203=DIRECTION('center_axis',(0.,-1.,0.));
#15204=DIRECTION('ref_axis',(-1.83697019872103E-16,0.,1.));
#15205=DIRECTION('center_axis',(0.,1.,0.));
#15206=DIRECTION('ref_axis',(1.,0.,0.));
#15207=DIRECTION('center_axis',(0.,-1.,0.));
#15208=DIRECTION('ref_axis',(0.309016994374947,0.,0.951056516295154));
#15209=DIRECTION('center_axis',(0.,1.,0.));
#15210=DIRECTION('ref_axis',(1.,0.,0.));
#15211=DIRECTION('center_axis',(0.,-1.,0.));
#15212=DIRECTION('ref_axis',(0.587785252292473,0.,0.809016994374948));
#15213=DIRECTION('center_axis',(0.,1.,0.));
#15214=DIRECTION('ref_axis',(1.,0.,0.));
#15215=DIRECTION('center_axis',(0.,-1.,0.));
#15216=DIRECTION('ref_axis',(0.809016994374947,0.,0.587785252292473));
#15217=DIRECTION('center_axis',(0.,1.,0.));
#15218=DIRECTION('ref_axis',(1.,0.,0.));
#15219=DIRECTION('center_axis',(0.,1.,0.));
#15220=DIRECTION('ref_axis',(1.,0.,0.));
#15221=DIRECTION('center_axis',(0.,1.,0.));
#15222=DIRECTION('ref_axis',(1.,0.,0.));
#15223=DIRECTION('',(0.,-1.,0.));
#15224=DIRECTION('center_axis',(0.,1.,0.));
#15225=DIRECTION('ref_axis',(1.,0.,0.));
#15226=DIRECTION('center_axis',(0.,1.,0.));
#15227=DIRECTION('ref_axis',(-0.951056516295153,0.,-0.309016994374948));
#15228=DIRECTION('',(0.,-1.,0.));
#15229=DIRECTION('',(0.,1.,0.));
#15230=DIRECTION('center_axis',(0.,1.,0.));
#15231=DIRECTION('ref_axis',(1.,0.,0.));
#15232=DIRECTION('',(0.,-1.,0.));
#15233=DIRECTION('center_axis',(0.,1.,0.));
#15234=DIRECTION('ref_axis',(-0.809016994374947,0.,-0.587785252292473));
#15235=DIRECTION('',(0.,1.,0.));
#15236=DIRECTION('center_axis',(0.,1.,0.));
#15237=DIRECTION('ref_axis',(1.,0.,0.));
#15238=DIRECTION('',(0.,-1.,0.));
#15239=DIRECTION('center_axis',(0.,1.,0.));
#15240=DIRECTION('ref_axis',(-0.587785252292473,0.,-0.809016994374947));
#15241=DIRECTION('',(0.,1.,0.));
#15242=DIRECTION('center_axis',(0.,1.,0.));
#15243=DIRECTION('ref_axis',(1.,0.,0.));
#15244=DIRECTION('',(0.,-1.,0.));
#15245=DIRECTION('center_axis',(0.,1.,0.));
#15246=DIRECTION('ref_axis',(-0.309016994374947,0.,-0.951056516295154));
#15247=DIRECTION('',(0.,1.,0.));
#15248=DIRECTION('center_axis',(0.,1.,0.));
#15249=DIRECTION('ref_axis',(1.,0.,0.));
#15250=DIRECTION('',(0.,-1.,0.));
#15251=DIRECTION('center_axis',(0.,1.,0.));
#15252=DIRECTION('ref_axis',(-1.37927510063224E-16,0.,-1.));
#15253=DIRECTION('',(0.,1.,0.));
#15254=DIRECTION('center_axis',(0.,1.,0.));
#15255=DIRECTION('ref_axis',(1.,0.,0.));
#15256=DIRECTION('',(0.,-1.,0.));
#15257=DIRECTION('center_axis',(0.,1.,0.));
#15258=DIRECTION('ref_axis',(0.309016994374948,0.,-0.951056516295154));
#15259=DIRECTION('',(0.,1.,0.));
#15260=DIRECTION('center_axis',(0.,1.,0.));
#15261=DIRECTION('ref_axis',(1.,0.,0.));
#15262=DIRECTION('',(0.,-1.,0.));
#15263=DIRECTION('center_axis',(0.,1.,0.));
#15264=DIRECTION('ref_axis',(0.587785252292473,0.,-0.809016994374948));
#15265=DIRECTION('',(0.,1.,0.));
#15266=DIRECTION('center_axis',(0.,1.,0.));
#15267=DIRECTION('ref_axis',(1.,0.,0.));
#15268=DIRECTION('',(0.,-1.,0.));
#15269=DIRECTION('center_axis',(0.,1.,0.));
#15270=DIRECTION('ref_axis',(0.809016994374948,0.,-0.587785252292473));
#15271=DIRECTION('',(0.,1.,0.));
#15272=DIRECTION('center_axis',(0.,1.,0.));
#15273=DIRECTION('ref_axis',(1.,0.,0.));
#15274=DIRECTION('',(0.,-1.,0.));
#15275=DIRECTION('center_axis',(0.,1.,0.));
#15276=DIRECTION('ref_axis',(0.951056516295154,0.,-0.309016994374947));
#15277=DIRECTION('',(0.,1.,0.));
#15278=DIRECTION('center_axis',(0.,1.,0.));
#15279=DIRECTION('ref_axis',(1.,0.,0.));
#15280=DIRECTION('',(0.,-1.,0.));
#15281=DIRECTION('center_axis',(0.,1.,0.));
#15282=DIRECTION('ref_axis',(1.,0.,-1.99159850020592E-16));
#15283=DIRECTION('',(0.,1.,0.));
#15284=DIRECTION('center_axis',(0.,1.,0.));
#15285=DIRECTION('ref_axis',(1.,0.,0.));
#15286=DIRECTION('',(0.,-1.,0.));
#15287=DIRECTION('center_axis',(0.,1.,0.));
#15288=DIRECTION('ref_axis',(0.951056516295154,0.,0.309016994374948));
#15289=DIRECTION('',(0.,1.,0.));
#15290=DIRECTION('center_axis',(0.,1.,0.));
#15291=DIRECTION('ref_axis',(1.,0.,0.));
#15292=DIRECTION('',(0.,-1.,0.));
#15293=DIRECTION('center_axis',(0.,1.,0.));
#15294=DIRECTION('ref_axis',(0.809016994374948,0.,0.587785252292473));
#15295=DIRECTION('',(0.,1.,0.));
#15296=DIRECTION('center_axis',(0.,1.,0.));
#15297=DIRECTION('ref_axis',(1.,0.,0.));
#15298=DIRECTION('',(0.,-1.,0.));
#15299=DIRECTION('center_axis',(0.,1.,0.));
#15300=DIRECTION('ref_axis',(0.587785252292473,0.,0.809016994374948));
#15301=DIRECTION('',(0.,1.,0.));
#15302=DIRECTION('center_axis',(0.,1.,0.));
#15303=DIRECTION('ref_axis',(1.,0.,0.));
#15304=DIRECTION('',(0.,-1.,0.));
#15305=DIRECTION('center_axis',(0.,1.,0.));
#15306=DIRECTION('ref_axis',(0.309016994374947,0.,0.951056516295154));
#15307=DIRECTION('',(0.,1.,0.));
#15308=DIRECTION('center_axis',(0.,1.,0.));
#15309=DIRECTION('ref_axis',(1.,0.,0.));
#15310=DIRECTION('',(0.,-1.,0.));
#15311=DIRECTION('center_axis',(0.,1.,0.));
#15312=DIRECTION('ref_axis',(2.6039218997796E-16,0.,1.));
#15313=DIRECTION('',(0.,1.,0.));
#15314=DIRECTION('center_axis',(0.,1.,0.));
#15315=DIRECTION('ref_axis',(1.,0.,0.));
#15316=DIRECTION('',(0.,-1.,0.));
#15317=DIRECTION('center_axis',(0.,1.,0.));
#15318=DIRECTION('ref_axis',(-0.309016994374948,0.,0.951056516295153));
#15319=DIRECTION('',(0.,1.,0.));
#15320=DIRECTION('center_axis',(0.,1.,0.));
#15321=DIRECTION('ref_axis',(1.,0.,0.));
#15322=DIRECTION('',(0.,-1.,0.));
#15323=DIRECTION('center_axis',(0.,1.,0.));
#15324=DIRECTION('ref_axis',(-0.587785252292474,0.,0.809016994374947));
#15325=DIRECTION('',(0.,1.,0.));
#15326=DIRECTION('center_axis',(0.,1.,0.));
#15327=DIRECTION('ref_axis',(1.,0.,0.));
#15328=DIRECTION('',(0.,-1.,0.));
#15329=DIRECTION('center_axis',(0.,1.,0.));
#15330=DIRECTION('ref_axis',(-0.809016994374948,0.,0.587785252292473));
#15331=DIRECTION('',(0.,1.,0.));
#15332=DIRECTION('center_axis',(0.,1.,0.));
#15333=DIRECTION('ref_axis',(1.,0.,0.));
#15334=DIRECTION('',(0.,-1.,0.));
#15335=DIRECTION('center_axis',(0.,1.,0.));
#15336=DIRECTION('ref_axis',(-0.951056516295154,0.,0.309016994374948));
#15337=DIRECTION('',(0.,1.,0.));
#15338=DIRECTION('center_axis',(0.,1.,0.));
#15339=DIRECTION('ref_axis',(1.,0.,0.));
#15340=DIRECTION('',(0.,1.,0.));
#15341=DIRECTION('center_axis',(0.,1.,0.));
#15342=DIRECTION('ref_axis',(-1.,0.,-1.22464679914735E-16));
#15343=DIRECTION('',(0.,-1.,0.));
#15344=DIRECTION('center_axis',(0.,1.,0.));
#15345=DIRECTION('ref_axis',(1.,0.,0.));
#18620=CARTESIAN_POINT('',(0.,0.,0.));
#18621=CARTESIAN_POINT('Origin',(0.,-0.45,0.));
#18622=CARTESIAN_POINT('',(-0.65,-0.325,-3.9801020972289E-17));
#18623=CARTESIAN_POINT('',(-0.637867541108654,-0.45,0.125));
#18624=CARTESIAN_POINT('Ctrl Pts',(-0.65,-0.325,-6.93889390390723E-17));
#18625=CARTESIAN_POINT('Ctrl Pts',(-0.65,-0.325,0.0157371373481997));
#18626=CARTESIAN_POINT('Ctrl Pts',(-0.649370620646074,-0.328153081062251,
0.0324967135411163));
#18627=CARTESIAN_POINT('Ctrl Pts',(-0.647096224417991,-0.340922081922822,
0.0632828231545122));
#18628=CARTESIAN_POINT('Ctrl Pts',(-0.645482573914132,-0.350535859112198,
0.0773125544088347));
#18629=CARTESIAN_POINT('Ctrl Pts',(-0.642442040715078,-0.372687974598127,
0.0994646698947638));
#18630=CARTESIAN_POINT('Ctrl Pts',(-0.640815160902589,-0.386717480603274,
0.109078032552995));
#18631=CARTESIAN_POINT('Ctrl Pts',(-0.63851034608138,-0.417502809542363,
0.121846732641678));
#18632=CARTESIAN_POINT('Ctrl Pts',(-0.637867541108654,-0.434262111007648,
0.125));
#18633=CARTESIAN_POINT('Ctrl Pts',(-0.637867541108654,-0.45,0.125));
#18634=CARTESIAN_POINT('',(-0.65,-0.575,-3.9801020972289E-17));
#18635=CARTESIAN_POINT('Ctrl Pts',(-0.65,-0.575,-3.46944695195361E-18));
#18636=CARTESIAN_POINT('Ctrl Pts',(-0.65,-0.575,-0.0157371373481998));
#18637=CARTESIAN_POINT('Ctrl Pts',(-0.649370620646074,-0.571846918937749,
-0.0324967135411164));
#18638=CARTESIAN_POINT('Ctrl Pts',(-0.647096224417991,-0.559077918077178,
-0.0632828231545123));
#18639=CARTESIAN_POINT('Ctrl Pts',(-0.645482573914132,-0.549464140887802,
-0.0773125544088349));
#18640=CARTESIAN_POINT('Ctrl Pts',(-0.642442040715078,-0.527312025401873,
-0.099464669894764));
#18641=CARTESIAN_POINT('Ctrl Pts',(-0.640815160902589,-0.513282519396725,
-0.109078032552995));
#18642=CARTESIAN_POINT('Ctrl Pts',(-0.63851034608138,-0.482497190457637,
-0.121846732641678));
#18643=CARTESIAN_POINT('Ctrl Pts',(-0.637867541108654,-0.465737888992352,
-0.125));
#18644=CARTESIAN_POINT('Ctrl Pts',(-0.637867541108654,-0.434262111007648,
-0.125));
#18645=CARTESIAN_POINT('Ctrl Pts',(-0.63851034608138,-0.417502809542363,
-0.121846732641678));
#18646=CARTESIAN_POINT('Ctrl Pts',(-0.640815160902589,-0.386717480603275,
-0.109078032552995));
#18647=CARTESIAN_POINT('Ctrl Pts',(-0.642442040715078,-0.372687974598127,
-0.099464669894764));
#18648=CARTESIAN_POINT('Ctrl Pts',(-0.645482573914132,-0.350535859112198,
-0.077312554408835));
#18649=CARTESIAN_POINT('Ctrl Pts',(-0.647096224417991,-0.340922081922822,
-0.0632828231545124));
#18650=CARTESIAN_POINT('Ctrl Pts',(-0.649370620646074,-0.328153081062251,
-0.0324967135411165));
#18651=CARTESIAN_POINT('Ctrl Pts',(-0.65,-0.325,-0.0157371373481999));
#18652=CARTESIAN_POINT('Ctrl Pts',(-0.65,-0.325,-8.32667268468867E-17));
#18653=CARTESIAN_POINT('Ctrl Pts',(-0.637867541108654,-0.45,0.125));
#18654=CARTESIAN_POINT('Ctrl Pts',(-0.637867541108654,-0.465737888992352,
0.125));
#18655=CARTESIAN_POINT('Ctrl Pts',(-0.63851034608138,-0.482497190457637,
0.121846732641678));
#18656=CARTESIAN_POINT('Ctrl Pts',(-0.640815160902589,-0.513282519396725,
0.109078032552995));
#18657=CARTESIAN_POINT('Ctrl Pts',(-0.642442040715078,-0.527312025401873,
0.0994646698947639));
#18658=CARTESIAN_POINT('Ctrl Pts',(-0.645482573914132,-0.549464140887802,
0.0773125544088349));
#18659=CARTESIAN_POINT('Ctrl Pts',(-0.647096224417991,-0.559077918077178,
0.0632828231545123));
#18660=CARTESIAN_POINT('Ctrl Pts',(-0.649370620646074,-0.571846918937749,
0.0324967135411164));
#18661=CARTESIAN_POINT('Ctrl Pts',(-0.65,-0.575,0.0157371373481998));
#18662=CARTESIAN_POINT('Ctrl Pts',(-0.65,-0.575,-2.08166817117217E-17));
#18663=CARTESIAN_POINT('',(-0.379967103839267,-0.45,0.125));
#18664=CARTESIAN_POINT('',(-7.65404249467096E-18,-0.45,0.125));
#18665=CARTESIAN_POINT('',(-0.4,-0.575,5.41097774720219E-18));
#18666=CARTESIAN_POINT('Ctrl Pts',(-0.4,-0.575,-3.81639164714898E-17));
#18667=CARTESIAN_POINT('Ctrl Pts',(-0.4,-0.575,0.0158075115832675));
#18668=CARTESIAN_POINT('Ctrl Pts',(-0.398970551469948,-0.571819306519379,
0.0325978607437828));
#18669=CARTESIAN_POINT('Ctrl Pts',(-0.395252954914593,-0.559029081159106,
0.0633657881355917));
#18670=CARTESIAN_POINT('Ctrl Pts',(-0.392612801026882,-0.549425200318011,
0.0773514949786256));
#18671=CARTESIAN_POINT('Ctrl Pts',(-0.38761064154154,-0.527347592689753,
0.0994291026068839));
#18672=CARTESIAN_POINT('Ctrl Pts',(-0.384911758361269,-0.51336346023721,
0.109029967924066));
#18673=CARTESIAN_POINT('Ctrl Pts',(-0.381057715344782,-0.48260129709332,
0.121817958968287));
#18674=CARTESIAN_POINT('Ctrl Pts',(-0.379967103839267,-0.465813100629203,
0.125));
#18675=CARTESIAN_POINT('Ctrl Pts',(-0.379967103839267,-0.45,0.125));
#18676=CARTESIAN_POINT('',(-0.379967103839267,-0.45,-0.125));
#18677=CARTESIAN_POINT('Ctrl Pts',(-0.379967103839267,-0.45,-0.125));
#18678=CARTESIAN_POINT('Ctrl Pts',(-0.379967103839267,-0.465813100629203,
-0.125));
#18679=CARTESIAN_POINT('Ctrl Pts',(-0.381057715344782,-0.48260129709332,
-0.121817958968287));
#18680=CARTESIAN_POINT('Ctrl Pts',(-0.384911758361269,-0.51336346023721,
-0.109029967924066));
#18681=CARTESIAN_POINT('Ctrl Pts',(-0.38761064154154,-0.527347592689753,
-0.099429102606884));
#18682=CARTESIAN_POINT('Ctrl Pts',(-0.392612801026882,-0.549425200318011,
-0.0773514949786257));
#18683=CARTESIAN_POINT('Ctrl Pts',(-0.395252954914593,-0.559029081159106,
-0.0633657881355918));
#18684=CARTESIAN_POINT('Ctrl Pts',(-0.398970551469948,-0.571819306519379,
-0.0325978607437828));
#18685=CARTESIAN_POINT('Ctrl Pts',(-0.4,-0.575,-0.0158075115832676));
#18686=CARTESIAN_POINT('Ctrl Pts',(-0.4,-0.575,-4.16333634234434E-17));
#18687=CARTESIAN_POINT('',(-0.4,-0.325,2.96971064108775E-17));
#18688=CARTESIAN_POINT('Ctrl Pts',(-0.4,-0.325,1.04083408558608E-17));
#18689=CARTESIAN_POINT('Ctrl Pts',(-0.4,-0.325,-0.0158075115832676));
#18690=CARTESIAN_POINT('Ctrl Pts',(-0.398970551469948,-0.328180693480621,
-0.0325978607437828));
#18691=CARTESIAN_POINT('Ctrl Pts',(-0.395252954914593,-0.340970918840894,
-0.0633657881355918));
#18692=CARTESIAN_POINT('Ctrl Pts',(-0.392612801026882,-0.350574799681989,
-0.0773514949786256));
#18693=CARTESIAN_POINT('Ctrl Pts',(-0.38761064154154,-0.372652407310247,
-0.0994291026068839));
#18694=CARTESIAN_POINT('Ctrl Pts',(-0.384911758361269,-0.38663653976279,
-0.109029967924066));
#18695=CARTESIAN_POINT('Ctrl Pts',(-0.381057715344782,-0.41739870290668,
-0.121817958968287));
#18696=CARTESIAN_POINT('Ctrl Pts',(-0.379967103839267,-0.434186899370797,
-0.125));
#18697=CARTESIAN_POINT('Ctrl Pts',(-0.379967103839267,-0.45,-0.125));
#18698=CARTESIAN_POINT('Ctrl Pts',(-0.379967103839267,-0.45,0.125));
#18699=CARTESIAN_POINT('Ctrl Pts',(-0.379967103839267,-0.434186899370797,
0.125));
#18700=CARTESIAN_POINT('Ctrl Pts',(-0.381057715344782,-0.41739870290668,
0.121817958968287));
#18701=CARTESIAN_POINT('Ctrl Pts',(-0.384911758361269,-0.38663653976279,
0.109029967924066));
#18702=CARTESIAN_POINT('Ctrl Pts',(-0.38761064154154,-0.372652407310247,
0.0994291026068839));
#18703=CARTESIAN_POINT('Ctrl Pts',(-0.392612801026882,-0.350574799681989,
0.0773514949786257));
#18704=CARTESIAN_POINT('Ctrl Pts',(-0.395252954914593,-0.340970918840894,
0.0633657881355918));
#18705=CARTESIAN_POINT('Ctrl Pts',(-0.398970551469948,-0.328180693480621,
0.0325978607437829));
#18706=CARTESIAN_POINT('Ctrl Pts',(-0.4,-0.325,0.0158075115832676));
#18707=CARTESIAN_POINT('Ctrl Pts',(-0.4,-0.325,1.38777878078145E-17));
#18708=CARTESIAN_POINT('Origin',(0.,-0.45,0.));
#18709=CARTESIAN_POINT('',(0.379967103839267,-0.45,-0.125));
#18710=CARTESIAN_POINT('',(0.379967103839267,-0.45,0.125));
#18711=CARTESIAN_POINT('Ctrl Pts',(0.379967103839267,-0.45,-0.125));
#18712=CARTESIAN_POINT('Ctrl Pts',(0.379967103839267,-0.434186899370797,
-0.125));
#18713=CARTESIAN_POINT('Ctrl Pts',(0.381057715344782,-0.41739870290668,
-0.121817958968287));
#18714=CARTESIAN_POINT('Ctrl Pts',(0.384911758361269,-0.38663653976279,
-0.109029967924066));
#18715=CARTESIAN_POINT('Ctrl Pts',(0.38761064154154,-0.372652407310247,
-0.0994291026068839));
#18716=CARTESIAN_POINT('Ctrl Pts',(0.392612801026882,-0.350574799681989,
-0.0773514949786256));
#18717=CARTESIAN_POINT('Ctrl Pts',(0.395252954914593,-0.340970918840894,
-0.0633657881355917));
#18718=CARTESIAN_POINT('Ctrl Pts',(0.398970551469948,-0.328180693480621,
-0.0325978607437828));
#18719=CARTESIAN_POINT('Ctrl Pts',(0.4,-0.325,-0.0158075115832675));
#18720=CARTESIAN_POINT('Ctrl Pts',(0.4,-0.325,0.0158075115832676));
#18721=CARTESIAN_POINT('Ctrl Pts',(0.398970551469948,-0.328180693480621,
0.0325978607437829));
#18722=CARTESIAN_POINT('Ctrl Pts',(0.395252954914593,-0.340970918840894,
0.0633657881355918));
#18723=CARTESIAN_POINT('Ctrl Pts',(0.392612801026882,-0.350574799681989,
0.0773514949786257));
#18724=CARTESIAN_POINT('Ctrl Pts',(0.38761064154154,-0.372652407310247,
0.099429102606884));
#18725=CARTESIAN_POINT('Ctrl Pts',(0.384911758361269,-0.38663653976279,
0.109029967924066));
#18726=CARTESIAN_POINT('Ctrl Pts',(0.381057715344782,-0.41739870290668,
0.121817958968287));
#18727=CARTESIAN_POINT('Ctrl Pts',(0.379967103839267,-0.434186899370797,
0.125));
#18728=CARTESIAN_POINT('Ctrl Pts',(0.379967103839267,-0.45,0.125));
#18729=CARTESIAN_POINT('Ctrl Pts',(0.379967103839267,-0.45,0.125));
#18730=CARTESIAN_POINT('Ctrl Pts',(0.379967103839267,-0.465813100629203,
0.125));
#18731=CARTESIAN_POINT('Ctrl Pts',(0.381057715344782,-0.48260129709332,
0.121817958968287));
#18732=CARTESIAN_POINT('Ctrl Pts',(0.384911758361269,-0.51336346023721,
0.109029967924066));
#18733=CARTESIAN_POINT('Ctrl Pts',(0.38761064154154,-0.527347592689753,
0.0994291026068839));
#18734=CARTESIAN_POINT('Ctrl Pts',(0.392612801026882,-0.549425200318011,
0.0773514949786257));
#18735=CARTESIAN_POINT('Ctrl Pts',(0.395252954914593,-0.559029081159106,
0.0633657881355918));
#18736=CARTESIAN_POINT('Ctrl Pts',(0.398970551469948,-0.571819306519379,
0.0325978607437829));
#18737=CARTESIAN_POINT('Ctrl Pts',(0.4,-0.575,0.0158075115832676));
#18738=CARTESIAN_POINT('Ctrl Pts',(0.4,-0.575,-0.0158075115832676));
#18739=CARTESIAN_POINT('Ctrl Pts',(0.398970551469948,-0.57181930651938,
-0.0325978607437828));
#18740=CARTESIAN_POINT('Ctrl Pts',(0.395252954914593,-0.559029081159106,
-0.0633657881355918));
#18741=CARTESIAN_POINT('Ctrl Pts',(0.392612801026882,-0.549425200318011,
-0.0773514949786257));
#18742=CARTESIAN_POINT('Ctrl Pts',(0.38761064154154,-0.527347592689753,
-0.0994291026068839));
#18743=CARTESIAN_POINT('Ctrl Pts',(0.384911758361269,-0.51336346023721,
-0.109029967924066));
#18744=CARTESIAN_POINT('Ctrl Pts',(0.381057715344782,-0.48260129709332,
-0.121817958968287));
#18745=CARTESIAN_POINT('Ctrl Pts',(0.379967103839267,-0.465813100629203,
-0.125));
#18746=CARTESIAN_POINT('Ctrl Pts',(0.379967103839267,-0.45,-0.125));
#18747=CARTESIAN_POINT('',(0.637867541108654,-0.45,0.125));
#18748=CARTESIAN_POINT('',(-7.65404249467096E-18,-0.45,0.125));
#18749=CARTESIAN_POINT('',(0.65,-0.575,3.9801020972289E-17));
#18750=CARTESIAN_POINT('Ctrl Pts',(0.65,-0.575,5.55111512312578E-17));
#18751=CARTESIAN_POINT('Ctrl Pts',(0.65,-0.575,0.0157371373481999));
#18752=CARTESIAN_POINT('Ctrl Pts',(0.649370620646074,-0.571846918937749,
0.0324967135411165));
#18753=CARTESIAN_POINT('Ctrl Pts',(0.647096224417991,-0.559077918077178,
0.0632828231545124));
#18754=CARTESIAN_POINT('Ctrl Pts',(0.645482573914132,-0.549464140887802,
0.077312554408835));
#18755=CARTESIAN_POINT('Ctrl Pts',(0.642442040715078,-0.527312025401873,
0.099464669894764));
#18756=CARTESIAN_POINT('Ctrl Pts',(0.640815160902589,-0.513282519396725,
0.109078032552995));
#18757=CARTESIAN_POINT('Ctrl Pts',(0.63851034608138,-0.482497190457637,
0.121846732641678));
#18758=CARTESIAN_POINT('Ctrl Pts',(0.637867541108654,-0.465737888992352,
0.125));
#18759=CARTESIAN_POINT('Ctrl Pts',(0.637867541108654,-0.45,0.125));
#18760=CARTESIAN_POINT('',(0.65,-0.325,3.9801020972289E-17));
#18761=CARTESIAN_POINT('Ctrl Pts',(0.65,-0.325,6.93889390390723E-18));
#18762=CARTESIAN_POINT('Ctrl Pts',(0.65,-0.325,-0.0157371373481998));
#18763=CARTESIAN_POINT('Ctrl Pts',(0.649370620646074,-0.328153081062251,
-0.0324967135411164));
#18764=CARTESIAN_POINT('Ctrl Pts',(0.647096224417991,-0.340922081922822,
-0.0632828231545123));
#18765=CARTESIAN_POINT('Ctrl Pts',(0.645482573914132,-0.350535859112198,
-0.0773125544088349));
#18766=CARTESIAN_POINT('Ctrl Pts',(0.642442040715078,-0.372687974598127,
-0.0994646698947639));
#18767=CARTESIAN_POINT('Ctrl Pts',(0.640815160902588,-0.386717480603275,
-0.109078032552995));
#18768=CARTESIAN_POINT('Ctrl Pts',(0.63851034608138,-0.417502809542363,
-0.121846732641678));
#18769=CARTESIAN_POINT('Ctrl Pts',(0.637867541108654,-0.434262111007648,
-0.125));
#18770=CARTESIAN_POINT('Ctrl Pts',(0.637867541108654,-0.465737888992352,
-0.125));
#18771=CARTESIAN_POINT('Ctrl Pts',(0.63851034608138,-0.482497190457637,
-0.121846732641678));
#18772=CARTESIAN_POINT('Ctrl Pts',(0.640815160902589,-0.513282519396725,
-0.109078032552995));
#18773=CARTESIAN_POINT('Ctrl Pts',(0.642442040715078,-0.527312025401873,
-0.0994646698947639));
#18774=CARTESIAN_POINT('Ctrl Pts',(0.645482573914132,-0.549464140887802,
-0.0773125544088348));
#18775=CARTESIAN_POINT('Ctrl Pts',(0.647096224417991,-0.559077918077178,
-0.0632828231545123));
#18776=CARTESIAN_POINT('Ctrl Pts',(0.649370620646074,-0.571846918937749,
-0.0324967135411164));
#18777=CARTESIAN_POINT('Ctrl Pts',(0.65,-0.575,-0.0157371373481998));
#18778=CARTESIAN_POINT('Ctrl Pts',(0.65,-0.575,6.24500451351651E-17));
#18779=CARTESIAN_POINT('Ctrl Pts',(0.637867541108654,-0.45,0.125));
#18780=CARTESIAN_POINT('Ctrl Pts',(0.637867541108654,-0.434262111007648,
0.125));
#18781=CARTESIAN_POINT('Ctrl Pts',(0.63851034608138,-0.417502809542363,
0.121846732641678));
#18782=CARTESIAN_POINT('Ctrl Pts',(0.640815160902589,-0.386717480603274,
0.109078032552995));
#18783=CARTESIAN_POINT('Ctrl Pts',(0.642442040715078,-0.372687974598127,
0.0994646698947639));
#18784=CARTESIAN_POINT('Ctrl Pts',(0.645482573914132,-0.350535859112198,
0.0773125544088348));
#18785=CARTESIAN_POINT('Ctrl Pts',(0.647096224417991,-0.340922081922822,
0.0632828231545123));
#18786=CARTESIAN_POINT('Ctrl Pts',(0.649370620646074,-0.328153081062251,
0.0324967135411164));
#18787=CARTESIAN_POINT('Ctrl Pts',(0.65,-0.325,0.0157371373481998));
#18788=CARTESIAN_POINT('Ctrl Pts',(0.65,-0.325,-6.93889390390723E-18));
#18789=CARTESIAN_POINT('Origin',(0.,-0.1,0.));
#18790=CARTESIAN_POINT('',(-0.65,-0.8,7.9602041944578E-17));
#18791=CARTESIAN_POINT('Origin',(0.,-0.8,0.));
#18792=CARTESIAN_POINT('',(-0.65,-0.1,-7.9602041944578E-17));
#18793=CARTESIAN_POINT('',(-0.65,-0.1,7.9602041944578E-17));
#18794=CARTESIAN_POINT('',(-0.65,-0.1,-7.9602041944578E-17));
#18795=CARTESIAN_POINT('Origin',(0.,-0.1,0.));
#18796=CARTESIAN_POINT('',(0.,-0.575,-0.65));
#18797=CARTESIAN_POINT('',(0.,-0.325,-0.65));
#18798=CARTESIAN_POINT('Ctrl Pts',(-1.73472347597681E-17,-0.575,-0.65));
#18799=CARTESIAN_POINT('Ctrl Pts',(0.0157371373481998,-0.575,-0.65));
#18800=CARTESIAN_POINT('Ctrl Pts',(0.0324967135411164,-0.571846918937749,
-0.649370620646074));
#18801=CARTESIAN_POINT('Ctrl Pts',(0.0632828231545123,-0.559077918077178,
-0.647096224417991));
#18802=CARTESIAN_POINT('Ctrl Pts',(0.0773125544088349,-0.549464140887802,
-0.645482573914132));
#18803=CARTESIAN_POINT('Ctrl Pts',(0.099464669894764,-0.527312025401873,
-0.642442040715078));
#18804=CARTESIAN_POINT('Ctrl Pts',(0.109078032552995,-0.513282519396725,
-0.640815160902589));
#18805=CARTESIAN_POINT('Ctrl Pts',(0.121846732641678,-0.482497190457636,
-0.63851034608138));
#18806=CARTESIAN_POINT('Ctrl Pts',(0.125,-0.465737888992352,-0.637867541108654));
#18807=CARTESIAN_POINT('Ctrl Pts',(0.125,-0.434262111007648,-0.637867541108654));
#18808=CARTESIAN_POINT('Ctrl Pts',(0.121846732641678,-0.417502809542364,
-0.63851034608138));
#18809=CARTESIAN_POINT('Ctrl Pts',(0.109078032552995,-0.386717480603275,
-0.640815160902589));
#18810=CARTESIAN_POINT('Ctrl Pts',(0.099464669894764,-0.372687974598127,
-0.642442040715078));
#18811=CARTESIAN_POINT('Ctrl Pts',(0.0773125544088349,-0.350535859112198,
-0.645482573914132));
#18812=CARTESIAN_POINT('Ctrl Pts',(0.0632828231545123,-0.340922081922822,
-0.647096224417991));
#18813=CARTESIAN_POINT('Ctrl Pts',(0.0324967135411164,-0.328153081062251,
-0.649370620646074));
#18814=CARTESIAN_POINT('Ctrl Pts',(0.0157371373481999,-0.325,-0.65));
#18815=CARTESIAN_POINT('Ctrl Pts',(4.5102810375397E-17,-0.325,-0.65));
#18816=CARTESIAN_POINT('',(-0.125,-0.45,-0.637867541108654));
#18817=CARTESIAN_POINT('Ctrl Pts',(4.85722573273506E-17,-0.325,-0.65));
#18818=CARTESIAN_POINT('Ctrl Pts',(-0.0157371373481997,-0.325,-0.65));
#18819=CARTESIAN_POINT('Ctrl Pts',(-0.0324967135411163,-0.328153081062251,
-0.649370620646074));
#18820=CARTESIAN_POINT('Ctrl Pts',(-0.0632828231545122,-0.340922081922822,
-0.647096224417991));
#18821=CARTESIAN_POINT('Ctrl Pts',(-0.0773125544088348,-0.350535859112198,
-0.645482573914132));
#18822=CARTESIAN_POINT('Ctrl Pts',(-0.0994646698947639,-0.372687974598127,
-0.642442040715078));
#18823=CARTESIAN_POINT('Ctrl Pts',(-0.109078032552995,-0.386717480603274,
-0.640815160902589));
#18824=CARTESIAN_POINT('Ctrl Pts',(-0.121846732641678,-0.417502809542363,
-0.63851034608138));
#18825=CARTESIAN_POINT('Ctrl Pts',(-0.125,-0.434262111007648,-0.637867541108654));
#18826=CARTESIAN_POINT('Ctrl Pts',(-0.125,-0.45,-0.637867541108654));
#18827=CARTESIAN_POINT('Ctrl Pts',(-0.125,-0.45,-0.637867541108654));
#18828=CARTESIAN_POINT('Ctrl Pts',(-0.125,-0.465737888992352,-0.637867541108654));
#18829=CARTESIAN_POINT('Ctrl Pts',(-0.121846732641678,-0.482497190457636,
-0.63851034608138));
#18830=CARTESIAN_POINT('Ctrl Pts',(-0.109078032552995,-0.513282519396725,
-0.640815160902589));
#18831=CARTESIAN_POINT('Ctrl Pts',(-0.099464669894764,-0.527312025401873,
-0.642442040715078));
#18832=CARTESIAN_POINT('Ctrl Pts',(-0.0773125544088349,-0.549464140887802,
-0.645482573914132));
#18833=CARTESIAN_POINT('Ctrl Pts',(-0.0632828231545124,-0.559077918077178,
-0.647096224417991));
#18834=CARTESIAN_POINT('Ctrl Pts',(-0.0324967135411165,-0.571846918937749,
-0.649370620646074));
#18835=CARTESIAN_POINT('Ctrl Pts',(-0.0157371373481998,-0.575,-0.65));
#18836=CARTESIAN_POINT('Ctrl Pts',(-1.73472347597681E-17,-0.575,-0.65));
#18837=CARTESIAN_POINT('',(0.,-0.325,0.65));
#18838=CARTESIAN_POINT('',(0.,-0.575,0.65));
#18839=CARTESIAN_POINT('Ctrl Pts',(2.77555756156289E-17,-0.325,0.65));
#18840=CARTESIAN_POINT('Ctrl Pts',(0.0157371373481998,-0.325,0.65));
#18841=CARTESIAN_POINT('Ctrl Pts',(0.0324967135411164,-0.328153081062251,
0.649370620646074));
#18842=CARTESIAN_POINT('Ctrl Pts',(0.0632828231545123,-0.340922081922822,
0.647096224417991));
#18843=CARTESIAN_POINT('Ctrl Pts',(0.0773125544088349,-0.350535859112198,
0.645482573914132));
#18844=CARTESIAN_POINT('Ctrl Pts',(0.099464669894764,-0.372687974598127,
0.642442040715078));
#18845=CARTESIAN_POINT('Ctrl Pts',(0.109078032552995,-0.386717480603275,
0.640815160902589));
#18846=CARTESIAN_POINT('Ctrl Pts',(0.121846732641678,-0.417502809542364,
0.63851034608138));
#18847=CARTESIAN_POINT('Ctrl Pts',(0.125,-0.434262111007648,0.637867541108654));
#18848=CARTESIAN_POINT('Ctrl Pts',(0.125,-0.465737888992352,0.637867541108654));
#18849=CARTESIAN_POINT('Ctrl Pts',(0.121846732641678,-0.482497190457636,
0.63851034608138));
#18850=CARTESIAN_POINT('Ctrl Pts',(0.109078032552995,-0.513282519396725,
0.640815160902589));
#18851=CARTESIAN_POINT('Ctrl Pts',(0.099464669894764,-0.527312025401873,
0.642442040715078));
#18852=CARTESIAN_POINT('Ctrl Pts',(0.077312554408835,-0.549464140887802,
0.645482573914132));
#18853=CARTESIAN_POINT('Ctrl Pts',(0.0632828231545124,-0.559077918077178,
0.647096224417991));
#18854=CARTESIAN_POINT('Ctrl Pts',(0.0324967135411165,-0.571846918937749,
0.649370620646074));
#18855=CARTESIAN_POINT('Ctrl Pts',(0.0157371373481998,-0.575,0.65));
#18856=CARTESIAN_POINT('Ctrl Pts',(-1.38777878078145E-17,-0.575,0.65));
#18857=CARTESIAN_POINT('',(-0.125,-0.45,0.637867541108654));
#18858=CARTESIAN_POINT('Ctrl Pts',(-1.04083408558608E-17,-0.575,0.65));
#18859=CARTESIAN_POINT('Ctrl Pts',(-0.0157371373481998,-0.575,0.65));
#18860=CARTESIAN_POINT('Ctrl Pts',(-0.0324967135411164,-0.571846918937749,
0.649370620646074));
#18861=CARTESIAN_POINT('Ctrl Pts',(-0.0632828231545123,-0.559077918077178,
0.647096224417991));
#18862=CARTESIAN_POINT('Ctrl Pts',(-0.0773125544088349,-0.549464140887802,
0.645482573914132));
#18863=CARTESIAN_POINT('Ctrl Pts',(-0.099464669894764,-0.527312025401873,
0.642442040715078));
#18864=CARTESIAN_POINT('Ctrl Pts',(-0.109078032552995,-0.513282519396725,
0.640815160902589));
#18865=CARTESIAN_POINT('Ctrl Pts',(-0.121846732641678,-0.482497190457636,
0.63851034608138));
#18866=CARTESIAN_POINT('Ctrl Pts',(-0.125,-0.465737888992352,0.637867541108654));
#18867=CARTESIAN_POINT('Ctrl Pts',(-0.125,-0.45,0.637867541108654));
#18868=CARTESIAN_POINT('Ctrl Pts',(-0.125,-0.45,0.637867541108654));
#18869=CARTESIAN_POINT('Ctrl Pts',(-0.125,-0.434262111007648,0.637867541108654));
#18870=CARTESIAN_POINT('Ctrl Pts',(-0.121846732641678,-0.417502809542363,
0.63851034608138));
#18871=CARTESIAN_POINT('Ctrl Pts',(-0.109078032552995,-0.386717480603274,
0.640815160902589));
#18872=CARTESIAN_POINT('Ctrl Pts',(-0.0994646698947639,-0.372687974598127,
0.642442040715078));
#18873=CARTESIAN_POINT('Ctrl Pts',(-0.0773125544088348,-0.350535859112198,
0.645482573914132));
#18874=CARTESIAN_POINT('Ctrl Pts',(-0.0632828231545122,-0.340922081922822,
0.647096224417991));
#18875=CARTESIAN_POINT('Ctrl Pts',(-0.0324967135411163,-0.328153081062251,
0.649370620646074));
#18876=CARTESIAN_POINT('Ctrl Pts',(-0.0157371373481998,-0.325,0.65));
#18877=CARTESIAN_POINT('Ctrl Pts',(4.5102810375397E-17,-0.325,0.65));
#18878=CARTESIAN_POINT('Origin',(0.,-0.45,0.));
#18879=CARTESIAN_POINT('',(-0.125,-0.45,-0.379967103839267));
#18880=CARTESIAN_POINT('',(-0.125,-0.45,0.));
#18881=CARTESIAN_POINT('',(0.125,-0.45,-0.379967103839267));
#18882=CARTESIAN_POINT('Ctrl Pts',(0.125,-0.45,-0.379967103839267));
#18883=CARTESIAN_POINT('Ctrl Pts',(0.125,-0.465813100629203,-0.379967103839267));
#18884=CARTESIAN_POINT('Ctrl Pts',(0.121817958968287,-0.48260129709332,
-0.381057715344782));
#18885=CARTESIAN_POINT('Ctrl Pts',(0.109029967924066,-0.51336346023721,
-0.384911758361269));
#18886=CARTESIAN_POINT('Ctrl Pts',(0.0994291026068839,-0.527347592689753,
-0.38761064154154));
#18887=CARTESIAN_POINT('Ctrl Pts',(0.0773514949786257,-0.549425200318011,
-0.392612801026882));
#18888=CARTESIAN_POINT('Ctrl Pts',(0.0633657881355918,-0.559029081159106,
-0.395252954914593));
#18889=CARTESIAN_POINT('Ctrl Pts',(0.0325978607437828,-0.571819306519379,
-0.398970551469948));
#18890=CARTESIAN_POINT('Ctrl Pts',(0.0158075115832676,-0.575,-0.4));
#18891=CARTESIAN_POINT('Ctrl Pts',(-0.0158075115832676,-0.575,-0.4));
#18892=CARTESIAN_POINT('Ctrl Pts',(-0.0325978607437828,-0.571819306519379,
-0.398970551469948));
#18893=CARTESIAN_POINT('Ctrl Pts',(-0.0633657881355918,-0.559029081159106,
-0.395252954914593));
#18894=CARTESIAN_POINT('Ctrl Pts',(-0.0773514949786256,-0.549425200318011,
-0.392612801026882));
#18895=CARTESIAN_POINT('Ctrl Pts',(-0.0994291026068839,-0.527347592689753,
-0.38761064154154));
#18896=CARTESIAN_POINT('Ctrl Pts',(-0.109029967924066,-0.51336346023721,
-0.384911758361269));
#18897=CARTESIAN_POINT('Ctrl Pts',(-0.121817958968287,-0.48260129709332,
-0.381057715344782));
#18898=CARTESIAN_POINT('Ctrl Pts',(-0.125,-0.465813100629203,-0.379967103839267));
#18899=CARTESIAN_POINT('Ctrl Pts',(-0.125,-0.45,-0.379967103839267));
#18900=CARTESIAN_POINT('Ctrl Pts',(-0.125,-0.45,-0.379967103839267));
#18901=CARTESIAN_POINT('Ctrl Pts',(-0.125,-0.434186899370797,-0.379967103839267));
#18902=CARTESIAN_POINT('Ctrl Pts',(-0.121817958968287,-0.41739870290668,
-0.381057715344782));
#18903=CARTESIAN_POINT('Ctrl Pts',(-0.109029967924066,-0.38663653976279,
-0.384911758361269));
#18904=CARTESIAN_POINT('Ctrl Pts',(-0.0994291026068839,-0.372652407310247,
-0.38761064154154));
#18905=CARTESIAN_POINT('Ctrl Pts',(-0.0773514949786257,-0.350574799681989,
-0.392612801026882));
#18906=CARTESIAN_POINT('Ctrl Pts',(-0.0633657881355918,-0.340970918840894,
-0.395252954914593));
#18907=CARTESIAN_POINT('Ctrl Pts',(-0.0325978607437829,-0.328180693480621,
-0.398970551469948));
#18908=CARTESIAN_POINT('Ctrl Pts',(-0.0158075115832676,-0.325,-0.4));
#18909=CARTESIAN_POINT('Ctrl Pts',(0.0158075115832675,-0.325,-0.4));
#18910=CARTESIAN_POINT('Ctrl Pts',(0.0325978607437828,-0.328180693480621,
-0.398970551469948));
#18911=CARTESIAN_POINT('Ctrl Pts',(0.0633657881355917,-0.340970918840894,
-0.395252954914593));
#18912=CARTESIAN_POINT('Ctrl Pts',(0.0773514949786256,-0.350574799681989,
-0.392612801026882));
#18913=CARTESIAN_POINT('Ctrl Pts',(0.0994291026068839,-0.372652407310247,
-0.38761064154154));
#18914=CARTESIAN_POINT('Ctrl Pts',(0.109029967924066,-0.38663653976279,
-0.384911758361269));
#18915=CARTESIAN_POINT('Ctrl Pts',(0.121817958968287,-0.41739870290668,
-0.381057715344782));
#18916=CARTESIAN_POINT('Ctrl Pts',(0.125,-0.434186899370797,-0.379967103839267));
#18917=CARTESIAN_POINT('Ctrl Pts',(0.125,-0.45,-0.379967103839267));
#18918=CARTESIAN_POINT('Origin',(0.,-0.45,0.));
#18919=CARTESIAN_POINT('',(0.125,-0.45,0.379967103839267));
#18920=CARTESIAN_POINT('',(-0.125,-0.45,0.379967103839267));
#18921=CARTESIAN_POINT('Ctrl Pts',(0.125,-0.45,0.379967103839267));
#18922=CARTESIAN_POINT('Ctrl Pts',(0.125,-0.434186899370797,0.379967103839267));
#18923=CARTESIAN_POINT('Ctrl Pts',(0.121817958968287,-0.41739870290668,
0.381057715344782));
#18924=CARTESIAN_POINT('Ctrl Pts',(0.109029967924066,-0.38663653976279,
0.384911758361269));
#18925=CARTESIAN_POINT('Ctrl Pts',(0.0994291026068839,-0.372652407310247,
0.38761064154154));
#18926=CARTESIAN_POINT('Ctrl Pts',(0.0773514949786256,-0.350574799681989,
0.392612801026882));
#18927=CARTESIAN_POINT('Ctrl Pts',(0.0633657881355918,-0.340970918840894,
0.395252954914593));
#18928=CARTESIAN_POINT('Ctrl Pts',(0.0325978607437828,-0.328180693480621,
0.398970551469948));
#18929=CARTESIAN_POINT('Ctrl Pts',(0.0158075115832676,-0.325,0.4));
#18930=CARTESIAN_POINT('Ctrl Pts',(-0.0158075115832676,-0.325,0.4));
#18931=CARTESIAN_POINT('Ctrl Pts',(-0.0325978607437828,-0.328180693480621,
0.398970551469948));
#18932=CARTESIAN_POINT('Ctrl Pts',(-0.0633657881355918,-0.340970918840894,
0.395252954914593));
#18933=CARTESIAN_POINT('Ctrl Pts',(-0.0773514949786257,-0.350574799681989,
0.392612801026882));
#18934=CARTESIAN_POINT('Ctrl Pts',(-0.0994291026068839,-0.372652407310247,
0.38761064154154));
#18935=CARTESIAN_POINT('Ctrl Pts',(-0.109029967924066,-0.38663653976279,
0.384911758361269));
#18936=CARTESIAN_POINT('Ctrl Pts',(-0.121817958968287,-0.41739870290668,
0.381057715344782));
#18937=CARTESIAN_POINT('Ctrl Pts',(-0.125,-0.434186899370797,0.379967103839267));
#18938=CARTESIAN_POINT('Ctrl Pts',(-0.125,-0.45,0.379967103839267));
#18939=CARTESIAN_POINT('Ctrl Pts',(-0.125,-0.45,0.379967103839267));
#18940=CARTESIAN_POINT('Ctrl Pts',(-0.125,-0.465813100629203,0.379967103839267));
#18941=CARTESIAN_POINT('Ctrl Pts',(-0.121817958968287,-0.48260129709332,
0.381057715344782));
#18942=CARTESIAN_POINT('Ctrl Pts',(-0.109029967924066,-0.51336346023721,
0.384911758361269));
#18943=CARTESIAN_POINT('Ctrl Pts',(-0.0994291026068839,-0.527347592689753,
0.38761064154154));
#18944=CARTESIAN_POINT('Ctrl Pts',(-0.0773514949786256,-0.549425200318011,
0.392612801026882));
#18945=CARTESIAN_POINT('Ctrl Pts',(-0.0633657881355917,-0.559029081159106,
0.395252954914593));
#18946=CARTESIAN_POINT('Ctrl Pts',(-0.0325978607437828,-0.571819306519379,
0.398970551469948));
#18947=CARTESIAN_POINT('Ctrl Pts',(-0.0158075115832675,-0.575,0.4));
#18948=CARTESIAN_POINT('Ctrl Pts',(0.0158075115832676,-0.575,0.4));
#18949=CARTESIAN_POINT('Ctrl Pts',(0.0325978607437828,-0.571819306519379,
0.398970551469948));
#18950=CARTESIAN_POINT('Ctrl Pts',(0.0633657881355917,-0.559029081159106,
0.395252954914593));
#18951=CARTESIAN_POINT('Ctrl Pts',(0.0773514949786257,-0.549425200318011,
0.392612801026882));
#18952=CARTESIAN_POINT('Ctrl Pts',(0.0994291026068839,-0.527347592689753,
0.38761064154154));
#18953=CARTESIAN_POINT('Ctrl Pts',(0.109029967924066,-0.51336346023721,
0.384911758361269));
#18954=CARTESIAN_POINT('Ctrl Pts',(0.121817958968287,-0.48260129709332,
0.381057715344782));
#18955=CARTESIAN_POINT('Ctrl Pts',(0.125,-0.465813100629203,0.379967103839267));
#18956=CARTESIAN_POINT('Ctrl Pts',(0.125,-0.45,0.379967103839267));
#18957=CARTESIAN_POINT('',(-0.125,-0.45,0.));
#18958=CARTESIAN_POINT('Origin',(0.,0.,0.));
#18959=CARTESIAN_POINT('',(-0.4,-0.8,4.89858719658941E-17));
#18960=CARTESIAN_POINT('Origin',(0.,-0.8,0.));
#18961=CARTESIAN_POINT('',(-0.4,0.,4.89858719658941E-17));
#18962=CARTESIAN_POINT('',(-0.4,0.85,-4.89858719658941E-17));
#18963=CARTESIAN_POINT('',(-0.4,0.,4.89858719658941E-17));
#18964=CARTESIAN_POINT('Origin',(0.,0.85,0.));
#18965=CARTESIAN_POINT('Origin',(0.,-0.8,0.));
#18966=CARTESIAN_POINT('Origin',(0.,0.,0.));
#18967=CARTESIAN_POINT('',(-0.8,0.,9.79717439317883E-17));
#18968=CARTESIAN_POINT('Origin',(0.,0.,0.));
#18969=CARTESIAN_POINT('',(0.595438916863769,0.,0.137993139022126));
#18970=CARTESIAN_POINT('',(0.562830534889751,0.,0.238351419397483));
#18971=CARTESIAN_POINT('Origin',(0.562758945330873,0.,0.182851465569258));
#18972=CARTESIAN_POINT('',(0.523653836874034,0.,0.315240018494132));
#18973=CARTESIAN_POINT('Origin',(0.,0.,0.));
#18974=CARTESIAN_POINT('',(0.461629008549572,0.,0.40060987082025));
#18975=CARTESIAN_POINT('Origin',(0.478711351753049,0.,0.347804155687524));
#18976=CARTESIAN_POINT('',(0.40060987082025,0.,0.461629008549572));
#18977=CARTESIAN_POINT('Origin',(0.,0.,0.));
#18978=CARTESIAN_POINT('',(0.315240018494132,0.,0.523653836874034));
#18979=CARTESIAN_POINT('Origin',(0.347804155687523,0.,0.478711351753049));
#18980=CARTESIAN_POINT('',(0.238351419397483,0.,0.562830534889751));
#18981=CARTESIAN_POINT('Origin',(0.,0.,0.));
#18982=CARTESIAN_POINT('',(0.137993139022126,0.,0.595438916863769));
#18983=CARTESIAN_POINT('Origin',(0.182851465569258,0.,0.562758945330873));
#18984=CARTESIAN_POINT('',(0.0527614703521001,0.,0.608938287003997));
#18985=CARTESIAN_POINT('Origin',(0.,0.,0.));
#18986=CARTESIAN_POINT('',(-0.0527614703521003,0.,0.608938287003997));
#18987=CARTESIAN_POINT('Origin',(-1.08697158783324E-16,0.,0.591719772367581));
#18988=CARTESIAN_POINT('',(-0.137993139022126,0.,0.595438916863769));
#18989=CARTESIAN_POINT('Origin',(0.,0.,0.));
#18990=CARTESIAN_POINT('',(-0.238351419397483,0.,0.562830534889751));
#18991=CARTESIAN_POINT('Origin',(-0.182851465569258,0.,0.562758945330873));
#18992=CARTESIAN_POINT('',(-0.315240018494132,0.,0.523653836874034));
#18993=CARTESIAN_POINT('Origin',(0.,0.,0.));
#18994=CARTESIAN_POINT('',(-0.40060987082025,0.,0.461629008549572));
#18995=CARTESIAN_POINT('Origin',(-0.347804155687524,0.,0.478711351753049));
#18996=CARTESIAN_POINT('',(-0.461629008549572,0.,0.40060987082025));
#18997=CARTESIAN_POINT('Origin',(0.,0.,0.));
#18998=CARTESIAN_POINT('',(-0.523653836874034,0.,0.315240018494132));
#18999=CARTESIAN_POINT('Origin',(-0.478711351753049,0.,0.347804155687524));
#19000=CARTESIAN_POINT('',(-0.562830534889751,0.,0.238351419397483));
#19001=CARTESIAN_POINT('Origin',(0.,0.,0.));
#19002=CARTESIAN_POINT('',(-0.595438916863769,0.,0.137993139022126));
#19003=CARTESIAN_POINT('Origin',(-0.562758945330873,0.,0.182851465569258));
#19004=CARTESIAN_POINT('',(-0.608938287003997,0.,0.0527614703521002));
#19005=CARTESIAN_POINT('Origin',(0.,0.,0.));
#19006=CARTESIAN_POINT('',(-0.608938287003997,0.,-0.0527614703521003));
#19007=CARTESIAN_POINT('Origin',(-0.591719772367581,0.,-7.24647725222159E-17));
#19008=CARTESIAN_POINT('',(-0.595438916863769,0.,-0.137993139022126));
#19009=CARTESIAN_POINT('Origin',(0.,0.,0.));
#19010=CARTESIAN_POINT('',(-0.562830534889751,0.,-0.238351419397483));
#19011=CARTESIAN_POINT('Origin',(-0.562758945330873,0.,-0.182851465569258));
#19012=CARTESIAN_POINT('',(-0.523653836874034,0.,-0.315240018494132));
#19013=CARTESIAN_POINT('Origin',(0.,0.,0.));
#19014=CARTESIAN_POINT('',(-0.461629008549572,0.,-0.40060987082025));
#19015=CARTESIAN_POINT('Origin',(-0.478711351753049,0.,-0.347804155687524));
#19016=CARTESIAN_POINT('',(-0.40060987082025,0.,-0.461629008549572));
#19017=CARTESIAN_POINT('Origin',(0.,0.,0.));
#19018=CARTESIAN_POINT('',(-0.315240018494132,0.,-0.523653836874034));
#19019=CARTESIAN_POINT('Origin',(-0.347804155687524,0.,-0.478711351753049));
#19020=CARTESIAN_POINT('',(-0.238351419397483,0.,-0.562830534889751));
#19021=CARTESIAN_POINT('Origin',(0.,0.,0.));
#19022=CARTESIAN_POINT('',(-0.137993139022126,0.,-0.595438916863769));
#19023=CARTESIAN_POINT('Origin',(-0.182851465569258,0.,-0.562758945330873));
#19024=CARTESIAN_POINT('',(-0.0527614703521002,0.,-0.608938287003997));
#19025=CARTESIAN_POINT('Origin',(0.,0.,0.));
#19026=CARTESIAN_POINT('',(0.0527614703521003,0.,-0.608938287003997));
#19027=CARTESIAN_POINT('Origin',(3.6232386261108E-17,0.,-0.591719772367581));
#19028=CARTESIAN_POINT('',(0.137993139022126,0.,-0.595438916863769));
#19029=CARTESIAN_POINT('Origin',(0.,0.,0.));
#19030=CARTESIAN_POINT('',(0.238351419397483,0.,-0.562830534889751));
#19031=CARTESIAN_POINT('Origin',(0.182851465569258,0.,-0.562758945330873));
#19032=CARTESIAN_POINT('',(0.315240018494132,0.,-0.523653836874034));
#19033=CARTESIAN_POINT('Origin',(0.,0.,0.));
#19034=CARTESIAN_POINT('',(0.40060987082025,0.,-0.461629008549572));
#19035=CARTESIAN_POINT('Origin',(0.347804155687524,0.,-0.478711351753049));
#19036=CARTESIAN_POINT('',(0.461629008549572,0.,-0.40060987082025));
#19037=CARTESIAN_POINT('Origin',(0.,0.,0.));
#19038=CARTESIAN_POINT('',(0.523653836874034,0.,-0.315240018494132));
#19039=CARTESIAN_POINT('Origin',(0.478711351753049,0.,-0.347804155687524));
#19040=CARTESIAN_POINT('',(0.562830534889751,0.,-0.238351419397483));
#19041=CARTESIAN_POINT('Origin',(0.,0.,0.));
#19042=CARTESIAN_POINT('',(0.595438916863769,0.,-0.137993139022126));
#19043=CARTESIAN_POINT('Origin',(0.562758945330873,0.,-0.182851465569258));
#19044=CARTESIAN_POINT('',(0.608938287003997,0.,-0.0527614703521001));
#19045=CARTESIAN_POINT('Origin',(0.,0.,0.));
#19046=CARTESIAN_POINT('',(0.608938287003997,0.,0.0527614703521001));
#19047=CARTESIAN_POINT('Origin',(0.591719772367581,0.,0.));
#19048=CARTESIAN_POINT('Origin',(0.,0.,0.));
#19049=CARTESIAN_POINT('Origin',(0.,0.,0.));
#19050=CARTESIAN_POINT('',(-0.8,-0.1,9.79717439317883E-17));
#19051=CARTESIAN_POINT('Origin',(0.,-0.1,0.));
#19052=CARTESIAN_POINT('',(-0.8,0.,-9.79717439317883E-17));
#19053=CARTESIAN_POINT('Origin',(0.,-0.1,0.));
#19054=CARTESIAN_POINT('Origin',(0.,0.75,0.));
#19055=CARTESIAN_POINT('',(-0.8,0.75,9.79717439317883E-17));
#19056=CARTESIAN_POINT('Origin',(0.,0.75,0.));
#19057=CARTESIAN_POINT('',(0.562830534889751,0.75,0.238351419397483));
#19058=CARTESIAN_POINT('',(0.595438916863769,0.75,0.137993139022126));
#19059=CARTESIAN_POINT('Origin',(0.562758945330873,0.75,0.182851465569258));
#19060=CARTESIAN_POINT('',(0.608938287003997,0.75,0.0527614703521002));
#19061=CARTESIAN_POINT('Origin',(0.,0.75,0.));
#19062=CARTESIAN_POINT('',(0.608938287003997,0.75,-0.0527614703521002));
#19063=CARTESIAN_POINT('Origin',(0.591719772367581,0.75,0.));
#19064=CARTESIAN_POINT('',(0.595438916863769,0.75,-0.137993139022126));
#19065=CARTESIAN_POINT('Origin',(0.,0.75,0.));
#19066=CARTESIAN_POINT('',(0.562830534889751,0.75,-0.238351419397483));
#19067=CARTESIAN_POINT('Origin',(0.562758945330873,0.75,-0.182851465569258));
#19068=CARTESIAN_POINT('',(0.523653836874034,0.75,-0.315240018494132));
#19069=CARTESIAN_POINT('Origin',(0.,0.75,0.));
#19070=CARTESIAN_POINT('',(0.461629008549572,0.75,-0.40060987082025));
#19071=CARTESIAN_POINT('Origin',(0.478711351753049,0.75,-0.347804155687524));
#19072=CARTESIAN_POINT('',(0.40060987082025,0.75,-0.461629008549572));
#19073=CARTESIAN_POINT('Origin',(0.,0.75,0.));
#19074=CARTESIAN_POINT('',(0.315240018494132,0.75,-0.523653836874034));
#19075=CARTESIAN_POINT('Origin',(0.347804155687524,0.75,-0.478711351753049));
#19076=CARTESIAN_POINT('',(0.238351419397483,0.75,-0.562830534889751));
#19077=CARTESIAN_POINT('Origin',(0.,0.75,0.));
#19078=CARTESIAN_POINT('',(0.137993139022126,0.75,-0.595438916863769));
#19079=CARTESIAN_POINT('Origin',(0.182851465569258,0.75,-0.562758945330873));
#19080=CARTESIAN_POINT('',(0.0527614703521003,0.75,-0.608938287003997));
#19081=CARTESIAN_POINT('Origin',(0.,0.75,0.));
#19082=CARTESIAN_POINT('',(-0.0527614703521002,0.75,-0.608938287003997));
#19083=CARTESIAN_POINT('Origin',(3.6232386261108E-17,0.75,-0.591719772367581));
#19084=CARTESIAN_POINT('',(-0.137993139022126,0.75,-0.595438916863769));
#19085=CARTESIAN_POINT('Origin',(0.,0.75,0.));
#19086=CARTESIAN_POINT('',(-0.238351419397483,0.75,-0.562830534889751));
#19087=CARTESIAN_POINT('Origin',(-0.182851465569258,0.75,-0.562758945330873));
#19088=CARTESIAN_POINT('',(-0.315240018494132,0.75,-0.523653836874034));
#19089=CARTESIAN_POINT('Origin',(0.,0.75,0.));
#19090=CARTESIAN_POINT('',(-0.40060987082025,0.75,-0.461629008549572));
#19091=CARTESIAN_POINT('Origin',(-0.347804155687524,0.75,-0.478711351753049));
#19092=CARTESIAN_POINT('',(-0.461629008549572,0.75,-0.40060987082025));
#19093=CARTESIAN_POINT('Origin',(0.,0.75,0.));
#19094=CARTESIAN_POINT('',(-0.523653836874034,0.75,-0.315240018494132));
#19095=CARTESIAN_POINT('Origin',(-0.478711351753049,0.75,-0.347804155687524));
#19096=CARTESIAN_POINT('',(-0.562830534889751,0.75,-0.238351419397483));
#19097=CARTESIAN_POINT('Origin',(0.,0.75,0.));
#19098=CARTESIAN_POINT('',(-0.595438916863769,0.75,-0.137993139022126));
#19099=CARTESIAN_POINT('Origin',(-0.562758945330873,0.75,-0.182851465569258));
#19100=CARTESIAN_POINT('',(-0.608938287003997,0.75,-0.0527614703521003));
#19101=CARTESIAN_POINT('Origin',(0.,0.75,0.));
#19102=CARTESIAN_POINT('',(-0.608938287003997,0.75,0.0527614703521002));
#19103=CARTESIAN_POINT('Origin',(-0.591719772367581,0.75,-7.24647725222159E-17));
#19104=CARTESIAN_POINT('',(-0.595438916863769,0.75,0.137993139022126));
#19105=CARTESIAN_POINT('Origin',(0.,0.75,0.));
#19106=CARTESIAN_POINT('',(-0.562830534889751,0.75,0.238351419397483));
#19107=CARTESIAN_POINT('Origin',(-0.562758945330873,0.75,0.182851465569258));
#19108=CARTESIAN_POINT('',(-0.523653836874034,0.75,0.315240018494132));
#19109=CARTESIAN_POINT('Origin',(0.,0.75,0.));
#19110=CARTESIAN_POINT('',(-0.461629008549572,0.75,0.40060987082025));
#19111=CARTESIAN_POINT('Origin',(-0.478711351753049,0.75,0.347804155687524));
#19112=CARTESIAN_POINT('',(-0.40060987082025,0.75,0.461629008549572));
#19113=CARTESIAN_POINT('Origin',(0.,0.75,0.));
#19114=CARTESIAN_POINT('',(-0.315240018494132,0.75,0.523653836874034));
#19115=CARTESIAN_POINT('Origin',(-0.347804155687524,0.75,0.478711351753049));
#19116=CARTESIAN_POINT('',(-0.238351419397483,0.75,0.562830534889751));
#19117=CARTESIAN_POINT('Origin',(0.,0.75,0.));
#19118=CARTESIAN_POINT('',(-0.137993139022126,0.75,0.595438916863769));
#19119=CARTESIAN_POINT('Origin',(-0.182851465569258,0.75,0.562758945330873));
#19120=CARTESIAN_POINT('',(-0.0527614703521003,0.75,0.608938287003997));
#19121=CARTESIAN_POINT('Origin',(0.,0.75,0.));
#19122=CARTESIAN_POINT('',(0.0527614703521001,0.75,0.608938287003997));
#19123=CARTESIAN_POINT('Origin',(-1.08697158783324E-16,0.75,0.591719772367581));
#19124=CARTESIAN_POINT('',(0.137993139022126,0.75,0.595438916863769));
#19125=CARTESIAN_POINT('Origin',(0.,0.75,0.));
#19126=CARTESIAN_POINT('',(0.238351419397483,0.75,0.562830534889751));
#19127=CARTESIAN_POINT('Origin',(0.182851465569258,0.75,0.562758945330873));
#19128=CARTESIAN_POINT('',(0.315240018494132,0.75,0.523653836874034));
#19129=CARTESIAN_POINT('Origin',(0.,0.75,0.));
#19130=CARTESIAN_POINT('',(0.40060987082025,0.75,0.461629008549572));
#19131=CARTESIAN_POINT('Origin',(0.347804155687523,0.75,0.478711351753049));
#19132=CARTESIAN_POINT('',(0.461629008549572,0.75,0.40060987082025));
#19133=CARTESIAN_POINT('Origin',(0.,0.75,0.));
#19134=CARTESIAN_POINT('',(0.523653836874034,0.75,0.315240018494132));
#19135=CARTESIAN_POINT('Origin',(0.478711351753049,0.75,0.347804155687524));
#19136=CARTESIAN_POINT('Origin',(0.,0.75,0.));
#19137=CARTESIAN_POINT('Origin',(0.,0.75,0.));
#19138=CARTESIAN_POINT('',(-0.8,0.85,9.79717439317883E-17));
#19139=CARTESIAN_POINT('Origin',(0.,0.85,0.));
#19140=CARTESIAN_POINT('',(-0.8,0.75,9.79717439317883E-17));
#19141=CARTESIAN_POINT('Origin',(0.,0.85,0.));
#19142=CARTESIAN_POINT('Origin',(0.562758945330873,0.,0.182851465569258));
#19143=CARTESIAN_POINT('',(0.595438916863769,0.,0.137993139022126));
#19144=CARTESIAN_POINT('',(0.562830534889751,0.,0.238351419397483));
#19145=CARTESIAN_POINT('Origin',(0.,0.,0.));
#19146=CARTESIAN_POINT('',(0.523653836874034,0.,0.315240018494132));
#19147=CARTESIAN_POINT('Origin',(0.478711351753049,0.,0.347804155687524));
#19148=CARTESIAN_POINT('',(0.461629008549572,0.,0.40060987082025));
#19149=CARTESIAN_POINT('Origin',(0.,0.,0.));
#19150=CARTESIAN_POINT('',(0.40060987082025,0.,0.461629008549572));
#19151=CARTESIAN_POINT('Origin',(0.347804155687523,0.,0.478711351753049));
#19152=CARTESIAN_POINT('',(0.315240018494132,0.,0.523653836874034));
#19153=CARTESIAN_POINT('Origin',(0.,0.,0.));
#19154=CARTESIAN_POINT('',(0.238351419397483,0.,0.562830534889751));
#19155=CARTESIAN_POINT('Origin',(0.182851465569258,0.,0.562758945330873));
#19156=CARTESIAN_POINT('',(0.137993139022126,0.,0.595438916863769));
#19157=CARTESIAN_POINT('Origin',(0.,0.,0.));
#19158=CARTESIAN_POINT('',(0.0527614703521,0.,0.608938287003997));
#19159=CARTESIAN_POINT('Origin',(-1.08697158783324E-16,0.,0.591719772367581));
#19160=CARTESIAN_POINT('',(-0.0527614703521002,0.,0.608938287003997));
#19161=CARTESIAN_POINT('Origin',(0.,0.,0.));
#19162=CARTESIAN_POINT('',(-0.137993139022126,0.,0.595438916863769));
#19163=CARTESIAN_POINT('Origin',(-0.182851465569258,0.,0.562758945330873));
#19164=CARTESIAN_POINT('',(-0.238351419397483,0.,0.562830534889751));
#19165=CARTESIAN_POINT('Origin',(0.,0.,0.));
#19166=CARTESIAN_POINT('',(-0.315240018494132,0.,0.523653836874034));
#19167=CARTESIAN_POINT('Origin',(-0.347804155687524,0.,0.478711351753049));
#19168=CARTESIAN_POINT('',(-0.40060987082025,0.,0.461629008549572));
#19169=CARTESIAN_POINT('Origin',(0.,0.,0.));
#19170=CARTESIAN_POINT('',(-0.461629008549572,0.,0.40060987082025));
#19171=CARTESIAN_POINT('Origin',(-0.478711351753049,0.,0.347804155687524));
#19172=CARTESIAN_POINT('',(-0.523653836874034,0.,0.315240018494132));
#19173=CARTESIAN_POINT('Origin',(0.,0.,0.));
#19174=CARTESIAN_POINT('',(-0.562830534889751,0.,0.238351419397483));
#19175=CARTESIAN_POINT('Origin',(-0.562758945330873,0.,0.182851465569258));
#19176=CARTESIAN_POINT('',(-0.595438916863769,0.,0.137993139022126));
#19177=CARTESIAN_POINT('Origin',(0.,0.,0.));
#19178=CARTESIAN_POINT('',(-0.608938287003997,0.,0.0527614703521));
#19179=CARTESIAN_POINT('Origin',(-0.591719772367581,0.,-7.24647725222159E-17));
#19180=CARTESIAN_POINT('',(-0.608938287003997,0.,-0.0527614703521002));
#19181=CARTESIAN_POINT('Origin',(0.,0.,0.));
#19182=CARTESIAN_POINT('',(-0.595438916863769,0.,-0.137993139022126));
#19183=CARTESIAN_POINT('Origin',(-0.562758945330873,0.,-0.182851465569258));
#19184=CARTESIAN_POINT('',(-0.562830534889751,0.,-0.238351419397483));
#19185=CARTESIAN_POINT('Origin',(0.,0.,0.));
#19186=CARTESIAN_POINT('',(-0.523653836874034,0.,-0.315240018494132));
#19187=CARTESIAN_POINT('Origin',(-0.478711351753049,0.,-0.347804155687524));
#19188=CARTESIAN_POINT('',(-0.461629008549572,0.,-0.40060987082025));
#19189=CARTESIAN_POINT('Origin',(0.,0.,0.));
#19190=CARTESIAN_POINT('',(-0.40060987082025,0.,-0.461629008549572));
#19191=CARTESIAN_POINT('Origin',(-0.347804155687524,0.,-0.478711351753049));
#19192=CARTESIAN_POINT('',(-0.315240018494132,0.,-0.523653836874034));
#19193=CARTESIAN_POINT('Origin',(0.,0.,0.));
#19194=CARTESIAN_POINT('',(-0.238351419397483,0.,-0.562830534889751));
#19195=CARTESIAN_POINT('Origin',(-0.182851465569258,0.,-0.562758945330873));
#19196=CARTESIAN_POINT('',(-0.137993139022126,0.,-0.595438916863769));
#19197=CARTESIAN_POINT('Origin',(0.,0.,0.));
#19198=CARTESIAN_POINT('',(-0.0527614703521,0.,-0.608938287003997));
#19199=CARTESIAN_POINT('Origin',(3.6232386261108E-17,0.,-0.591719772367581));
#19200=CARTESIAN_POINT('',(0.0527614703521001,0.,-0.608938287003997));
#19201=CARTESIAN_POINT('Origin',(0.,0.,0.));
#19202=CARTESIAN_POINT('',(0.137993139022126,0.,-0.595438916863769));
#19203=CARTESIAN_POINT('Origin',(0.182851465569258,0.,-0.562758945330873));
#19204=CARTESIAN_POINT('',(0.238351419397483,0.,-0.562830534889751));
#19205=CARTESIAN_POINT('Origin',(0.,0.,0.));
#19206=CARTESIAN_POINT('',(0.315240018494132,0.,-0.523653836874034));
#19207=CARTESIAN_POINT('Origin',(0.347804155687524,0.,-0.478711351753049));
#19208=CARTESIAN_POINT('',(0.40060987082025,0.,-0.461629008549572));
#19209=CARTESIAN_POINT('Origin',(0.,0.,0.));
#19210=CARTESIAN_POINT('',(0.461629008549572,0.,-0.40060987082025));
#19211=CARTESIAN_POINT('Origin',(0.478711351753049,0.,-0.347804155687524));
#19212=CARTESIAN_POINT('',(0.523653836874034,0.,-0.315240018494132));
#19213=CARTESIAN_POINT('Origin',(0.,0.,0.));
#19214=CARTESIAN_POINT('',(0.562830534889751,0.,-0.238351419397483));
#19215=CARTESIAN_POINT('Origin',(0.562758945330873,0.,-0.182851465569258));
#19216=CARTESIAN_POINT('',(0.595438916863769,0.,-0.137993139022126));
#19217=CARTESIAN_POINT('Origin',(0.,0.,0.));
#19218=CARTESIAN_POINT('',(0.608938287003997,0.,0.0527614703521001));
#19219=CARTESIAN_POINT('Origin',(0.591719772367581,0.,0.));
#19220=CARTESIAN_POINT('',(0.608938287003997,0.,-0.0527614703521001));
#19221=CARTESIAN_POINT('Origin',(0.,0.,0.));
#20029=UNCERTAINTY_MEASURE_WITH_UNIT(LENGTH_MEASURE(0.001),#20097,
'DISTANCE_ACCURACY_VALUE',
'Maximum model space distance between geometric entities at asserted c
onnectivities');
#20042=UNCERTAINTY_MEASURE_WITH_UNIT(LENGTH_MEASURE(0.001),#20097,
'DISTANCE_ACCURACY_VALUE',
'Maximum model space distance between geometric entities at asserted c
onnectivities');
#20083=(
GEOMETRIC_REPRESENTATION_CONTEXT(3)
GLOBAL_UNCERTAINTY_ASSIGNED_CONTEXT((#20029))
GLOBAL_UNIT_ASSIGNED_CONTEXT((#20097,#20099,#20100))
REPRESENTATION_CONTEXT('','3D')
);
#20096=(
GEOMETRIC_REPRESENTATION_CONTEXT(3)
GLOBAL_UNCERTAINTY_ASSIGNED_CONTEXT((#20042))
GLOBAL_UNIT_ASSIGNED_CONTEXT((#20097,#20099,#20100))
REPRESENTATION_CONTEXT('','3D')
);
#20097=(
LENGTH_UNIT()
NAMED_UNIT(*)
SI_UNIT(.CENTI.,.METRE.)
);
#20099=(
NAMED_UNIT(*)
PLANE_ANGLE_UNIT()
SI_UNIT($,.RADIAN.)
);
#20100=(
NAMED_UNIT(*)
SI_UNIT($,.STERADIAN.)
SOLID_ANGLE_UNIT()
);
#20141=SHAPE_DEFINITION_REPRESENTATION(#20199,#20352);
#20199=PRODUCT_DEFINITION_SHAPE('',$,#20406);
#20352=SHAPE_REPRESENTATION('',(#12320),#20083);
#20365=PRODUCT_DEFINITION_CONTEXT('part definition',#20526,'design');
#20406=PRODUCT_DEFINITION(
'Timing Pulley - 2 mm Pitch, 20 Teeth, 8 mm Bore',
'Timing Pulley - 2 mm Pitch, 20 Teeth, 8 mm Bore',#20459,#20365);
#20459=PRODUCT_DEFINITION_FORMATION('',$,#20568);
#20526=APPLICATION_CONTEXT(
'Core Data for Automotive Mechanical Design Process');
#20527=PRODUCT_CONTEXT('part definition',#20526,'mechanical');
#20568=PRODUCT('Timing Pulley - 2 mm Pitch, 20 Teeth, 8 mm Bore',
'Timing Pulley - 2 mm Pitch, 20 Teeth, 8 mm Bore',
'Timing Pulley - 2 mm Pitch, 20 Teeth, 8 mm Bore',(#20527));
#20658=COLOUR_RGB('Off White',0.89,0.88,0.83);
#20659=FILL_AREA_STYLE_COLOUR('',#20658);
#20660=FILL_AREA_STYLE('',(#20659));
#20661=SURFACE_STYLE_FILL_AREA(#20660);
#20662=SURFACE_SIDE_STYLE('',(#20661));
#20663=SURFACE_STYLE_USAGE(.BOTH.,#20662);
#20664=PRESENTATION_STYLE_ASSIGNMENT((#20663));
ENDSEC;
END-ISO-10303-21;
